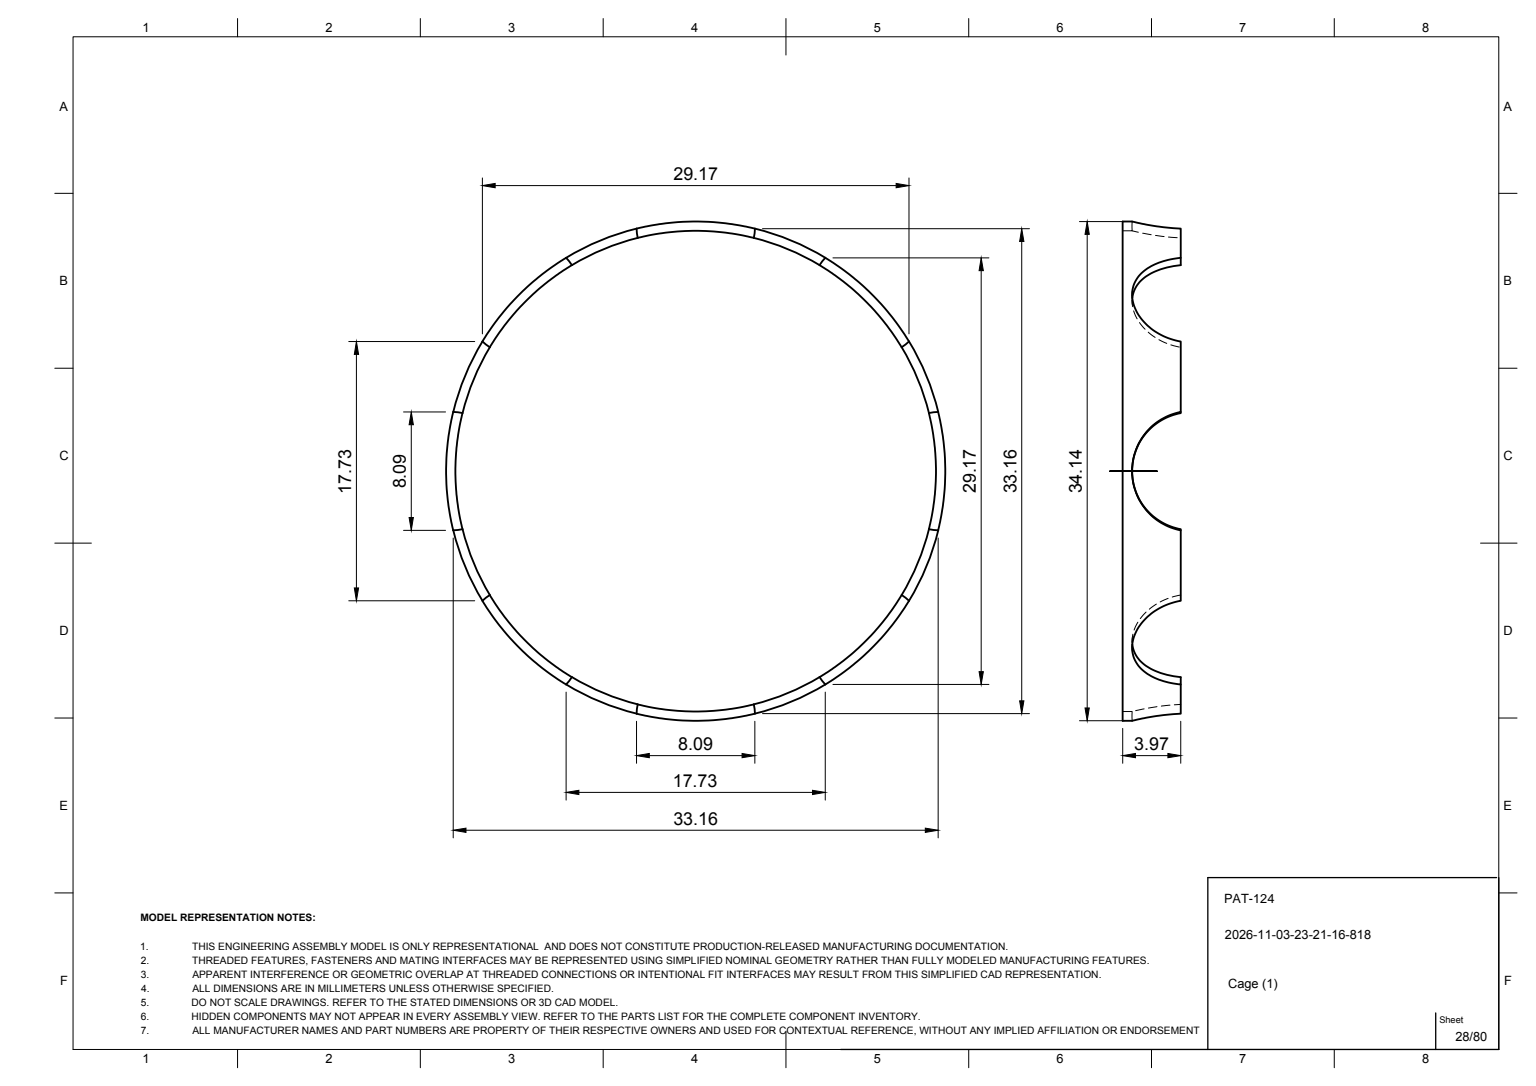
ISO-10303-21;
HEADER;
/* Generated by software containing ST-Developer
 * from STEP Tools, Inc. (www.steptools.com) 
 */

FILE_DESCRIPTION(
/* description */ ('XY cross-slide table'),
/* implementation_level */ '2;1');

FILE_NAME(
/* name */ 'Cage (1).step',
/* time_stamp */ '2026-10-28T03:22:46-07:00',
/* author */ (''),
/* organization */ (''),
/* preprocessor_version */ 'ST-DEVELOPER v20.2',
/* originating_system */ 'Autodesk Translation Framework v15.17.0.0',
/* authorisation */ '');

FILE_SCHEMA (('AUTOMOTIVE_DESIGN { 1 0 10303 214 3 1 1 }'));
ENDSEC;

DATA;
#10=MECHANICAL_DESIGN_GEOMETRIC_PRESENTATION_REPRESENTATION('',(#1703),#62984);
#707=B_SPLINE_CURVE_WITH_KNOTS('',3,(#34204,#34205,#34206,#34207,#34208,
#34209,#34210,#34211,#34212,#34213,#34214,#34215,#34216,#34217,#34218,#34219,
#34220,#34221,#34222,#34223,#34224,#34225),.UNSPECIFIED.,.F.,.F.,(4,2,2,
2,2,2,2,2,2,2,4),(0.0789094028588958,0.210573405340968,0.315860108011452,
0.421146810681936,0.522142632548711,0.623138454415485,0.72413427628226,
0.825130098149035,0.930416800819519,1.03570350349,1.16736750597208),
 .UNSPECIFIED.);
#708=B_SPLINE_CURVE_WITH_KNOTS('',3,(#34229,#34230,#34231,#34232,#34233,
#34234,#34235,#34236,#34237,#34238,#34239,#34240,#34241,#34242,#34243,#34244,
#34245,#34246,#34247,#34248,#34249,#34250),.UNSPECIFIED.,.F.,.F.,(4,2,2,
2,2,2,2,2,2,2,4),(0.0774793363974613,0.142088896491891,0.284177792983782,
0.411119756996526,0.514392970548519,0.617666184100513,0.720939397652506,
0.8242126112045,0.951154575217244,1.09324347170913,1.15785303180356),
 .UNSPECIFIED.);
#709=B_SPLINE_CURVE_WITH_KNOTS('',3,(#34256,#34257,#34258,#34259,#34260,
#34261,#34262,#34263,#34264,#34265,#34266,#34267,#34268,#34269,#34270,#34271,
#34272,#34273,#34274,#34275,#34276,#34277),.UNSPECIFIED.,.F.,.F.,(4,2,2,
2,2,2,2,2,2,2,4),(0.0774793363974613,0.142088896491891,0.284177792983782,
0.411119756996525,0.514392970548519,0.617666184100513,0.720939397652506,
0.8242126112045,0.951154575217243,1.09324347170913,1.15785303180356),
 .UNSPECIFIED.);
#710=B_SPLINE_CURVE_WITH_KNOTS('',3,(#34281,#34282,#34283,#34284,#34285,
#34286,#34287,#34288,#34289,#34290,#34291,#34292,#34293,#34294,#34295,#34296,
#34297,#34298,#34299,#34300,#34301,#34302),.UNSPECIFIED.,.F.,.F.,(4,2,2,
2,2,2,2,2,2,2,4),(0.0774793363974614,0.142088896491891,0.284177792983781,
0.411119756996525,0.514392970548519,0.617666184100512,0.720939397652506,
0.824212611204499,0.951154575217243,1.09324347170913,1.15785303180356),
 .UNSPECIFIED.);
#711=B_SPLINE_CURVE_WITH_KNOTS('',3,(#34306,#34307,#34308,#34309,#34310,
#34311,#34312,#34313,#34314,#34315,#34316,#34317),.UNSPECIFIED.,.F.,.F.,
(4,2,2,2,2,4),(0.0774793363974613,0.142088896491891,0.284177792983781,0.411119756996525,
0.514392970548519,0.617666184100512),.UNSPECIFIED.);
#712=B_SPLINE_CURVE_WITH_KNOTS('',3,(#34322,#34323,#34324,#34325,#34326,
#34327,#34328,#34329,#34330,#34331,#34332,#34333),.UNSPECIFIED.,.F.,.F.,
(4,2,2,2,2,4),(0.617666184100512,0.720939397652506,0.824212611204499,0.951154575217243,
1.09324347170913,1.15785303180356),.UNSPECIFIED.);
#713=B_SPLINE_CURVE_WITH_KNOTS('',3,(#34337,#34338,#34339,#34340,#34341,
#34342,#34343,#34344,#34345,#34346,#34347,#34348,#34349,#34350,#34351,#34352,
#34353,#34354,#34355,#34356,#34357,#34358),.UNSPECIFIED.,.F.,.F.,(4,2,2,
2,2,2,2,2,2,2,4),(0.0774793363974613,0.142088896491891,0.284177792983782,
0.411119756996526,0.514392970548519,0.617666184100513,0.720939397652507,
0.8242126112045,0.951154575217245,1.09324347170914,1.15785303180356),
 .UNSPECIFIED.);
#714=B_SPLINE_CURVE_WITH_KNOTS('',3,(#34362,#34363,#34364,#34365,#34366,
#34367,#34368,#34369,#34370,#34371,#34372,#34373,#34374,#34375,#34376,#34377,
#34378,#34379,#34380,#34381,#34382,#34383),.UNSPECIFIED.,.F.,.F.,(4,2,2,
2,2,2,2,2,2,2,4),(0.0774793363974613,0.142088896491891,0.284177792983782,
0.411119756996526,0.514392970548519,0.617666184100513,0.720939397652506,
0.824212611204499,0.951154575217243,1.09324347170913,1.15785303180356),
 .UNSPECIFIED.);
#715=B_SPLINE_CURVE_WITH_KNOTS('',3,(#34387,#34388,#34389,#34390,#34391,
#34392,#34393,#34394,#34395,#34396,#34397,#34398,#34399,#34400,#34401,#34402,
#34403,#34404,#34405,#34406,#34407,#34408),.UNSPECIFIED.,.F.,.F.,(4,2,2,
2,2,2,2,2,2,2,4),(0.0774793363974613,0.142088896491891,0.284177792983782,
0.411119756996526,0.514392970548519,0.617666184100513,0.720939397652506,
0.8242126112045,0.951154575217244,1.09324347170913,1.15785303180356),
 .UNSPECIFIED.);
#716=B_SPLINE_CURVE_WITH_KNOTS('',3,(#34412,#34413,#34414,#34415,#34416,
#34417,#34418,#34419,#34420,#34421,#34422,#34423,#34424,#34425,#34426,#34427,
#34428,#34429,#34430,#34431,#34432,#34433),.UNSPECIFIED.,.F.,.F.,(4,2,2,
2,2,2,2,2,2,2,4),(0.0774793363974613,0.142088896491891,0.284177792983782,
0.411119756996526,0.514392970548519,0.617666184100513,0.720939397652506,
0.8242126112045,0.951154575217243,1.09324347170913,1.15785303180356),
 .UNSPECIFIED.);
#717=B_SPLINE_CURVE_WITH_KNOTS('',3,(#34441,#34442,#34443,#34444,#34445,
#34446,#34447,#34448,#34449,#34450,#34451,#34452,#34453,#34454,#34455,#34456,
#34457,#34458,#34459,#34460,#34461,#34462),.UNSPECIFIED.,.F.,.F.,(4,2,2,
2,2,2,2,2,2,2,4),(0.0789094028588958,0.210573405340968,0.315860108011452,
0.421146810681936,0.522142632548711,0.623138454415485,0.72413427628226,
0.825130098149035,0.930416800819519,1.03570350349,1.16736750597208),
 .UNSPECIFIED.);
#718=B_SPLINE_CURVE_WITH_KNOTS('',3,(#34470,#34471,#34472,#34473,#34474,
#34475,#34476,#34477,#34478,#34479,#34480,#34481,#34482,#34483,#34484,#34485,
#34486,#34487,#34488,#34489,#34490,#34491),.UNSPECIFIED.,.F.,.F.,(4,2,2,
2,2,2,2,2,2,2,4),(0.0789094028588958,0.210573405340969,0.315860108011453,
0.421146810681937,0.522142632548712,0.623138454415486,0.724134276282261,
0.825130098149035,0.930416800819519,1.03570350349,1.16736750597208),
 .UNSPECIFIED.);
#719=B_SPLINE_CURVE_WITH_KNOTS('',3,(#34500,#34501,#34502,#34503,#34504,
#34505,#34506,#34507,#34508,#34509,#34510,#34511),.UNSPECIFIED.,.F.,.F.,
(4,2,2,2,2,4),(0.0789094028588958,0.210573405340968,0.315860108011452,0.421146810681937,
0.522142632548711,0.623138454415486),.UNSPECIFIED.);
#720=B_SPLINE_CURVE_WITH_KNOTS('',3,(#34513,#34514,#34515,#34516,#34517,
#34518,#34519,#34520,#34521,#34522,#34523,#34524),.UNSPECIFIED.,.F.,.F.,
(4,2,2,2,2,4),(0.623138454415486,0.72413427628226,0.825130098149035,0.930416800819519,
1.03570350349,1.16736750597208),.UNSPECIFIED.);
#721=B_SPLINE_CURVE_WITH_KNOTS('',3,(#34531,#34532,#34533,#34534,#34535,
#34536,#34537,#34538,#34539,#34540,#34541,#34542,#34543,#34544,#34545,#34546,
#34547,#34548,#34549,#34550,#34551,#34552),.UNSPECIFIED.,.F.,.F.,(4,2,2,
2,2,2,2,2,2,2,4),(0.0789094028588958,0.210573405340968,0.315860108011452,
0.421146810681936,0.522142632548711,0.623138454415486,0.72413427628226,
0.825130098149035,0.930416800819519,1.03570350349,1.16736750597208),
 .UNSPECIFIED.);
#722=B_SPLINE_CURVE_WITH_KNOTS('',3,(#34560,#34561,#34562,#34563,#34564,
#34565,#34566,#34567,#34568,#34569,#34570,#34571,#34572,#34573,#34574,#34575,
#34576,#34577,#34578,#34579,#34580,#34581),.UNSPECIFIED.,.F.,.F.,(4,2,2,
2,2,2,2,2,2,2,4),(0.0789094028588957,0.210573405340968,0.315860108011452,
0.421146810681936,0.522142632548711,0.623138454415485,0.72413427628226,
0.825130098149035,0.930416800819519,1.03570350349,1.16736750597207),
 .UNSPECIFIED.);
#723=B_SPLINE_CURVE_WITH_KNOTS('',3,(#34589,#34590,#34591,#34592,#34593,
#34594,#34595,#34596,#34597,#34598,#34599,#34600,#34601,#34602,#34603,#34604,
#34605,#34606,#34607,#34608,#34609,#34610),.UNSPECIFIED.,.F.,.F.,(4,2,2,
2,2,2,2,2,2,2,4),(0.0789094028588958,0.210573405340968,0.315860108011452,
0.421146810681936,0.522142632548711,0.623138454415486,0.72413427628226,
0.825130098149035,0.930416800819519,1.03570350349,1.16736750597208),
 .UNSPECIFIED.);
#724=B_SPLINE_CURVE_WITH_KNOTS('',3,(#34619,#34620,#34621,#34622,#34623,
#34624,#34625,#34626,#34627,#34628,#34629,#34630,#34631,#34632,#34633,#34634,
#34635,#34636,#34637,#34638,#34639,#34640),.UNSPECIFIED.,.F.,.F.,(4,2,2,
2,2,2,2,2,2,2,4),(0.0789094028588958,0.210573405340968,0.315860108011452,
0.421146810681936,0.522142632548711,0.623138454415485,0.72413427628226,
0.825130098149035,0.930416800819519,1.03570350349,1.16736750597208),
 .UNSPECIFIED.);
#1403=SPHERICAL_SURFACE('',#24472,0.412776);
#1404=SPHERICAL_SURFACE('',#24488,0.412776);
#1405=SPHERICAL_SURFACE('',#24493,0.412776);
#1406=SPHERICAL_SURFACE('',#24498,0.412776);
#1407=SPHERICAL_SURFACE('',#24503,0.412776);
#1408=SPHERICAL_SURFACE('',#24508,0.412776);
#1409=SPHERICAL_SURFACE('',#24513,0.412776);
#1410=SPHERICAL_SURFACE('',#24521,0.412776);
#1523=SHAPE_REPRESENTATION_RELATIONSHIP('SRR','None',#63373,#1606);
#1606=ADVANCED_BREP_SHAPE_REPRESENTATION('',(#1816),#62910);
#1703=STYLED_ITEM('',(#63912),#1816);
#1816=MANIFOLD_SOLID_BREP('Continuous crown cage',#22997);
#1996=FACE_BOUND('',#4529,.T.);
#2401=PLANE('',#24485);
#2402=PLANE('',#24490);
#2403=PLANE('',#24495);
#2404=PLANE('',#24500);
#2405=PLANE('',#24505);
#2406=PLANE('',#24510);
#2407=PLANE('',#24519);
#2408=PLANE('',#24523);
#2409=PLANE('',#24524);
#3088=FACE_OUTER_BOUND('',#4511,.T.);
#3089=FACE_OUTER_BOUND('',#4512,.T.);
#3090=FACE_OUTER_BOUND('',#4513,.T.);
#3091=FACE_OUTER_BOUND('',#4514,.T.);
#3092=FACE_OUTER_BOUND('',#4515,.T.);
#3093=FACE_OUTER_BOUND('',#4516,.T.);
#3094=FACE_OUTER_BOUND('',#4517,.T.);
#3095=FACE_OUTER_BOUND('',#4518,.T.);
#3096=FACE_OUTER_BOUND('',#4519,.T.);
#3097=FACE_OUTER_BOUND('',#4520,.T.);
#3098=FACE_OUTER_BOUND('',#4521,.T.);
#3099=FACE_OUTER_BOUND('',#4522,.T.);
#3100=FACE_OUTER_BOUND('',#4523,.T.);
#3101=FACE_OUTER_BOUND('',#4524,.T.);
#3102=FACE_OUTER_BOUND('',#4525,.T.);
#3103=FACE_OUTER_BOUND('',#4526,.T.);
#3104=FACE_OUTER_BOUND('',#4527,.T.);
#3105=FACE_OUTER_BOUND('',#4528,.T.);
#3106=FACE_OUTER_BOUND('',#4530,.T.);
#4511=EDGE_LOOP('',(#15832,#15833,#15834,#15835));
#4512=EDGE_LOOP('',(#15836,#15837,#15838,#15839,#15840,#15841,#15842,#15843,
#15844,#15845,#15846,#15847,#15848,#15849,#15850,#15851,#15852,#15853,#15854,
#15855));
#4513=EDGE_LOOP('',(#15856,#15857,#15858,#15859));
#4514=EDGE_LOOP('',(#15860,#15861,#15862,#15863));
#4515=EDGE_LOOP('',(#15864,#15865,#15866,#15867));
#4516=EDGE_LOOP('',(#15868,#15869,#15870,#15871));
#4517=EDGE_LOOP('',(#15872,#15873,#15874,#15875));
#4518=EDGE_LOOP('',(#15876,#15877,#15878,#15879,#15880,#15881));
#4519=EDGE_LOOP('',(#15882,#15883,#15884,#15885));
#4520=EDGE_LOOP('',(#15886,#15887,#15888,#15889));
#4521=EDGE_LOOP('',(#15890,#15891,#15892,#15893));
#4522=EDGE_LOOP('',(#15894,#15895,#15896,#15897));
#4523=EDGE_LOOP('',(#15898,#15899,#15900,#15901));
#4524=EDGE_LOOP('',(#15902,#15903,#15904,#15905));
#4525=EDGE_LOOP('',(#15906,#15907,#15908,#15909,#15910,#15911,#15912,#15913,
#15914,#15915,#15916,#15917,#15918,#15919,#15920,#15921,#15922,#15923,#15924,
#15925));
#4526=EDGE_LOOP('',(#15926,#15927,#15928,#15929));
#4527=EDGE_LOOP('',(#15930,#15931,#15932,#15933));
#4528=EDGE_LOOP('',(#15934));
#4529=EDGE_LOOP('',(#15935));
#4530=EDGE_LOOP('',(#15936,#15937,#15938,#15939));
#6133=LINE('',#34319,#7620);
#6134=LINE('',#34615,#7621);
#7620=VECTOR('',#27646,1.706752);
#7621=VECTOR('',#27723,1.643248);
#9103=CIRCLE('',#24473,0.405071403305639);
#9104=CIRCLE('',#24474,0.405071403305639);
#9105=CIRCLE('',#24476,1.706752);
#9106=CIRCLE('',#24477,1.706752);
#9107=CIRCLE('',#24478,1.706752);
#9108=CIRCLE('',#24479,1.706752);
#9109=CIRCLE('',#24480,1.706752);
#9110=CIRCLE('',#24481,1.706752);
#9111=CIRCLE('',#24482,1.706752);
#9112=CIRCLE('',#24483,1.706752);
#9113=CIRCLE('',#24484,1.706752);
#9114=CIRCLE('',#24486,1.643248);
#9115=CIRCLE('',#24487,0.405071403305639);
#9116=CIRCLE('',#24489,0.405071403305639);
#9117=CIRCLE('',#24491,1.643248);
#9118=CIRCLE('',#24492,0.405071403305639);
#9119=CIRCLE('',#24494,0.405071403305639);
#9120=CIRCLE('',#24496,1.643248);
#9121=CIRCLE('',#24497,0.405071403305639);
#9122=CIRCLE('',#24499,0.405071403305639);
#9123=CIRCLE('',#24501,1.643248);
#9124=CIRCLE('',#24502,0.405071403305639);
#9125=CIRCLE('',#24504,0.405071403305639);
#9126=CIRCLE('',#24506,1.643248);
#9127=CIRCLE('',#24507,0.405071403305639);
#9128=CIRCLE('',#24509,0.405071403305639);
#9129=CIRCLE('',#24511,1.643248);
#9130=CIRCLE('',#24512,0.405071403305639);
#9131=CIRCLE('',#24514,0.405071403305639);
#9132=CIRCLE('',#24516,1.643248);
#9133=CIRCLE('',#24517,1.643248);
#9134=CIRCLE('',#24518,1.643248);
#9135=CIRCLE('',#24520,0.405071403305639);
#9136=CIRCLE('',#24522,0.405071403305639);
#10097=VERTEX_POINT('',#34202);
#10098=VERTEX_POINT('',#34203);
#10099=VERTEX_POINT('',#34226);
#10100=VERTEX_POINT('',#34228);
#10101=VERTEX_POINT('',#34253);
#10102=VERTEX_POINT('',#34255);
#10103=VERTEX_POINT('',#34278);
#10104=VERTEX_POINT('',#34280);
#10105=VERTEX_POINT('',#34303);
#10106=VERTEX_POINT('',#34305);
#10107=VERTEX_POINT('',#34318);
#10108=VERTEX_POINT('',#34321);
#10109=VERTEX_POINT('',#34334);
#10110=VERTEX_POINT('',#34336);
#10111=VERTEX_POINT('',#34359);
#10112=VERTEX_POINT('',#34361);
#10113=VERTEX_POINT('',#34384);
#10114=VERTEX_POINT('',#34386);
#10115=VERTEX_POINT('',#34409);
#10116=VERTEX_POINT('',#34411);
#10117=VERTEX_POINT('',#34436);
#10118=VERTEX_POINT('',#34440);
#10119=VERTEX_POINT('',#34465);
#10120=VERTEX_POINT('',#34469);
#10121=VERTEX_POINT('',#34494);
#10122=VERTEX_POINT('',#34498);
#10123=VERTEX_POINT('',#34499);
#10124=VERTEX_POINT('',#34526);
#10125=VERTEX_POINT('',#34530);
#10126=VERTEX_POINT('',#34555);
#10127=VERTEX_POINT('',#34559);
#10128=VERTEX_POINT('',#34584);
#10129=VERTEX_POINT('',#34588);
#10130=VERTEX_POINT('',#34613);
#10131=VERTEX_POINT('',#34616);
#10132=VERTEX_POINT('',#34618);
#12300=EDGE_CURVE('',#10097,#10098,#707,.T.);
#12301=EDGE_CURVE('',#10099,#10097,#9103,.T.);
#12302=EDGE_CURVE('',#10100,#10099,#708,.T.);
#12303=EDGE_CURVE('',#10098,#10100,#9104,.T.);
#12304=EDGE_CURVE('',#10101,#10099,#9105,.T.);
#12305=EDGE_CURVE('',#10101,#10102,#709,.T.);
#12306=EDGE_CURVE('',#10103,#10102,#9106,.T.);
#12307=EDGE_CURVE('',#10103,#10104,#710,.T.);
#12308=EDGE_CURVE('',#10105,#10104,#9107,.T.);
#12309=EDGE_CURVE('',#10105,#10106,#711,.T.);
#12310=EDGE_CURVE('',#10106,#10107,#6133,.T.);
#12311=EDGE_CURVE('',#10107,#10107,#9108,.T.);
#12312=EDGE_CURVE('',#10106,#10108,#712,.T.);
#12313=EDGE_CURVE('',#10109,#10108,#9109,.T.);
#12314=EDGE_CURVE('',#10109,#10110,#713,.T.);
#12315=EDGE_CURVE('',#10111,#10110,#9110,.T.);
#12316=EDGE_CURVE('',#10111,#10112,#714,.T.);
#12317=EDGE_CURVE('',#10113,#10112,#9111,.T.);
#12318=EDGE_CURVE('',#10113,#10114,#715,.T.);
#12319=EDGE_CURVE('',#10115,#10114,#9112,.T.);
#12320=EDGE_CURVE('',#10115,#10116,#716,.T.);
#12321=EDGE_CURVE('',#10100,#10116,#9113,.T.);
#12322=EDGE_CURVE('',#10097,#10117,#9114,.T.);
#12323=EDGE_CURVE('',#10117,#10101,#9115,.T.);
#12324=EDGE_CURVE('',#10118,#10117,#717,.T.);
#12325=EDGE_CURVE('',#10102,#10118,#9116,.T.);
#12326=EDGE_CURVE('',#10118,#10119,#9117,.T.);
#12327=EDGE_CURVE('',#10119,#10103,#9118,.T.);
#12328=EDGE_CURVE('',#10120,#10119,#718,.T.);
#12329=EDGE_CURVE('',#10104,#10120,#9119,.T.);
#12330=EDGE_CURVE('',#10120,#10121,#9120,.T.);
#12331=EDGE_CURVE('',#10121,#10105,#9121,.T.);
#12332=EDGE_CURVE('',#10122,#10123,#719,.T.);
#12333=EDGE_CURVE('',#10108,#10122,#9122,.T.);
#12334=EDGE_CURVE('',#10123,#10121,#720,.T.);
#12335=EDGE_CURVE('',#10122,#10124,#9123,.T.);
#12336=EDGE_CURVE('',#10124,#10109,#9124,.T.);
#12337=EDGE_CURVE('',#10125,#10124,#721,.T.);
#12338=EDGE_CURVE('',#10110,#10125,#9125,.T.);
#12339=EDGE_CURVE('',#10125,#10126,#9126,.T.);
#12340=EDGE_CURVE('',#10126,#10111,#9127,.T.);
#12341=EDGE_CURVE('',#10127,#10126,#722,.T.);
#12342=EDGE_CURVE('',#10112,#10127,#9128,.T.);
#12343=EDGE_CURVE('',#10127,#10128,#9129,.T.);
#12344=EDGE_CURVE('',#10128,#10113,#9130,.T.);
#12345=EDGE_CURVE('',#10129,#10128,#723,.T.);
#12346=EDGE_CURVE('',#10114,#10129,#9131,.T.);
#12347=EDGE_CURVE('',#10130,#10130,#9132,.T.);
#12348=EDGE_CURVE('',#10130,#10123,#6134,.T.);
#12349=EDGE_CURVE('',#10131,#10098,#9133,.T.);
#12350=EDGE_CURVE('',#10131,#10132,#724,.T.);
#12351=EDGE_CURVE('',#10129,#10132,#9134,.T.);
#12352=EDGE_CURVE('',#10116,#10131,#9135,.T.);
#12353=EDGE_CURVE('',#10132,#10115,#9136,.T.);
#15832=ORIENTED_EDGE('',*,*,#12300,.F.);
#15833=ORIENTED_EDGE('',*,*,#12301,.F.);
#15834=ORIENTED_EDGE('',*,*,#12302,.F.);
#15835=ORIENTED_EDGE('',*,*,#12303,.F.);
#15836=ORIENTED_EDGE('',*,*,#12302,.T.);
#15837=ORIENTED_EDGE('',*,*,#12304,.F.);
#15838=ORIENTED_EDGE('',*,*,#12305,.T.);
#15839=ORIENTED_EDGE('',*,*,#12306,.F.);
#15840=ORIENTED_EDGE('',*,*,#12307,.T.);
#15841=ORIENTED_EDGE('',*,*,#12308,.F.);
#15842=ORIENTED_EDGE('',*,*,#12309,.T.);
#15843=ORIENTED_EDGE('',*,*,#12310,.T.);
#15844=ORIENTED_EDGE('',*,*,#12311,.F.);
#15845=ORIENTED_EDGE('',*,*,#12310,.F.);
#15846=ORIENTED_EDGE('',*,*,#12312,.T.);
#15847=ORIENTED_EDGE('',*,*,#12313,.F.);
#15848=ORIENTED_EDGE('',*,*,#12314,.T.);
#15849=ORIENTED_EDGE('',*,*,#12315,.F.);
#15850=ORIENTED_EDGE('',*,*,#12316,.T.);
#15851=ORIENTED_EDGE('',*,*,#12317,.F.);
#15852=ORIENTED_EDGE('',*,*,#12318,.T.);
#15853=ORIENTED_EDGE('',*,*,#12319,.F.);
#15854=ORIENTED_EDGE('',*,*,#12320,.T.);
#15855=ORIENTED_EDGE('',*,*,#12321,.F.);
#15856=ORIENTED_EDGE('',*,*,#12301,.T.);
#15857=ORIENTED_EDGE('',*,*,#12322,.T.);
#15858=ORIENTED_EDGE('',*,*,#12323,.T.);
#15859=ORIENTED_EDGE('',*,*,#12304,.T.);
#15860=ORIENTED_EDGE('',*,*,#12324,.F.);
#15861=ORIENTED_EDGE('',*,*,#12325,.F.);
#15862=ORIENTED_EDGE('',*,*,#12305,.F.);
#15863=ORIENTED_EDGE('',*,*,#12323,.F.);
#15864=ORIENTED_EDGE('',*,*,#12325,.T.);
#15865=ORIENTED_EDGE('',*,*,#12326,.T.);
#15866=ORIENTED_EDGE('',*,*,#12327,.T.);
#15867=ORIENTED_EDGE('',*,*,#12306,.T.);
#15868=ORIENTED_EDGE('',*,*,#12328,.F.);
#15869=ORIENTED_EDGE('',*,*,#12329,.F.);
#15870=ORIENTED_EDGE('',*,*,#12307,.F.);
#15871=ORIENTED_EDGE('',*,*,#12327,.F.);
#15872=ORIENTED_EDGE('',*,*,#12329,.T.);
#15873=ORIENTED_EDGE('',*,*,#12330,.T.);
#15874=ORIENTED_EDGE('',*,*,#12331,.T.);
#15875=ORIENTED_EDGE('',*,*,#12308,.T.);
#15876=ORIENTED_EDGE('',*,*,#12332,.F.);
#15877=ORIENTED_EDGE('',*,*,#12333,.F.);
#15878=ORIENTED_EDGE('',*,*,#12312,.F.);
#15879=ORIENTED_EDGE('',*,*,#12309,.F.);
#15880=ORIENTED_EDGE('',*,*,#12331,.F.);
#15881=ORIENTED_EDGE('',*,*,#12334,.F.);
#15882=ORIENTED_EDGE('',*,*,#12333,.T.);
#15883=ORIENTED_EDGE('',*,*,#12335,.T.);
#15884=ORIENTED_EDGE('',*,*,#12336,.T.);
#15885=ORIENTED_EDGE('',*,*,#12313,.T.);
#15886=ORIENTED_EDGE('',*,*,#12337,.F.);
#15887=ORIENTED_EDGE('',*,*,#12338,.F.);
#15888=ORIENTED_EDGE('',*,*,#12314,.F.);
#15889=ORIENTED_EDGE('',*,*,#12336,.F.);
#15890=ORIENTED_EDGE('',*,*,#12338,.T.);
#15891=ORIENTED_EDGE('',*,*,#12339,.T.);
#15892=ORIENTED_EDGE('',*,*,#12340,.T.);
#15893=ORIENTED_EDGE('',*,*,#12315,.T.);
#15894=ORIENTED_EDGE('',*,*,#12341,.F.);
#15895=ORIENTED_EDGE('',*,*,#12342,.F.);
#15896=ORIENTED_EDGE('',*,*,#12316,.F.);
#15897=ORIENTED_EDGE('',*,*,#12340,.F.);
#15898=ORIENTED_EDGE('',*,*,#12342,.T.);
#15899=ORIENTED_EDGE('',*,*,#12343,.T.);
#15900=ORIENTED_EDGE('',*,*,#12344,.T.);
#15901=ORIENTED_EDGE('',*,*,#12317,.T.);
#15902=ORIENTED_EDGE('',*,*,#12318,.F.);
#15903=ORIENTED_EDGE('',*,*,#12344,.F.);
#15904=ORIENTED_EDGE('',*,*,#12345,.F.);
#15905=ORIENTED_EDGE('',*,*,#12346,.F.);
#15906=ORIENTED_EDGE('',*,*,#12347,.F.);
#15907=ORIENTED_EDGE('',*,*,#12348,.T.);
#15908=ORIENTED_EDGE('',*,*,#12334,.T.);
#15909=ORIENTED_EDGE('',*,*,#12330,.F.);
#15910=ORIENTED_EDGE('',*,*,#12328,.T.);
#15911=ORIENTED_EDGE('',*,*,#12326,.F.);
#15912=ORIENTED_EDGE('',*,*,#12324,.T.);
#15913=ORIENTED_EDGE('',*,*,#12322,.F.);
#15914=ORIENTED_EDGE('',*,*,#12300,.T.);
#15915=ORIENTED_EDGE('',*,*,#12349,.F.);
#15916=ORIENTED_EDGE('',*,*,#12350,.T.);
#15917=ORIENTED_EDGE('',*,*,#12351,.F.);
#15918=ORIENTED_EDGE('',*,*,#12345,.T.);
#15919=ORIENTED_EDGE('',*,*,#12343,.F.);
#15920=ORIENTED_EDGE('',*,*,#12341,.T.);
#15921=ORIENTED_EDGE('',*,*,#12339,.F.);
#15922=ORIENTED_EDGE('',*,*,#12337,.T.);
#15923=ORIENTED_EDGE('',*,*,#12335,.F.);
#15924=ORIENTED_EDGE('',*,*,#12332,.T.);
#15925=ORIENTED_EDGE('',*,*,#12348,.F.);
#15926=ORIENTED_EDGE('',*,*,#12303,.T.);
#15927=ORIENTED_EDGE('',*,*,#12321,.T.);
#15928=ORIENTED_EDGE('',*,*,#12352,.T.);
#15929=ORIENTED_EDGE('',*,*,#12349,.T.);
#15930=ORIENTED_EDGE('',*,*,#12320,.F.);
#15931=ORIENTED_EDGE('',*,*,#12353,.F.);
#15932=ORIENTED_EDGE('',*,*,#12350,.F.);
#15933=ORIENTED_EDGE('',*,*,#12352,.F.);
#15934=ORIENTED_EDGE('',*,*,#12311,.T.);
#15935=ORIENTED_EDGE('',*,*,#12347,.T.);
#15936=ORIENTED_EDGE('',*,*,#12346,.T.);
#15937=ORIENTED_EDGE('',*,*,#12351,.T.);
#15938=ORIENTED_EDGE('',*,*,#12353,.T.);
#15939=ORIENTED_EDGE('',*,*,#12319,.T.);
#21120=CYLINDRICAL_SURFACE('',#24475,1.706752);
#21121=CYLINDRICAL_SURFACE('',#24515,1.643248);
#21869=ADVANCED_FACE('',(#3088),#1403,.F.);
#21870=ADVANCED_FACE('',(#3089),#21120,.T.);
#21871=ADVANCED_FACE('',(#3090),#2401,.T.);
#21872=ADVANCED_FACE('',(#3091),#1404,.F.);
#21873=ADVANCED_FACE('',(#3092),#2402,.T.);
#21874=ADVANCED_FACE('',(#3093),#1405,.F.);
#21875=ADVANCED_FACE('',(#3094),#2403,.T.);
#21876=ADVANCED_FACE('',(#3095),#1406,.F.);
#21877=ADVANCED_FACE('',(#3096),#2404,.T.);
#21878=ADVANCED_FACE('',(#3097),#1407,.F.);
#21879=ADVANCED_FACE('',(#3098),#2405,.T.);
#21880=ADVANCED_FACE('',(#3099),#1408,.F.);
#21881=ADVANCED_FACE('',(#3100),#2406,.T.);
#21882=ADVANCED_FACE('',(#3101),#1409,.F.);
#21883=ADVANCED_FACE('',(#3102),#21121,.F.);
#21884=ADVANCED_FACE('',(#3103),#2407,.T.);
#21885=ADVANCED_FACE('',(#3104),#1410,.F.);
#21886=ADVANCED_FACE('',(#3105,#1996),#2408,.T.);
#21887=ADVANCED_FACE('',(#3106),#2409,.T.);
#22997=CLOSED_SHELL('',(#21869,#21870,#21871,#21872,#21873,#21874,#21875,
#21876,#21877,#21878,#21879,#21880,#21881,#21882,#21883,#21884,#21885,#21886,
#21887));
#24471=AXIS2_PLACEMENT_3D('',#34200,#27630,#27631);
#24472=AXIS2_PLACEMENT_3D('',#34201,#27632,#27633);
#24473=AXIS2_PLACEMENT_3D('',#34227,#27634,#27635);
#24474=AXIS2_PLACEMENT_3D('',#34251,#27636,#27637);
#24475=AXIS2_PLACEMENT_3D('',#34252,#27638,#27639);
#24476=AXIS2_PLACEMENT_3D('',#34254,#27640,#27641);
#24477=AXIS2_PLACEMENT_3D('',#34279,#27642,#27643);
#24478=AXIS2_PLACEMENT_3D('',#34304,#27644,#27645);
#24479=AXIS2_PLACEMENT_3D('',#34320,#27647,#27648);
#24480=AXIS2_PLACEMENT_3D('',#34335,#27649,#27650);
#24481=AXIS2_PLACEMENT_3D('',#34360,#27651,#27652);
#24482=AXIS2_PLACEMENT_3D('',#34385,#27653,#27654);
#24483=AXIS2_PLACEMENT_3D('',#34410,#27655,#27656);
#24484=AXIS2_PLACEMENT_3D('',#34434,#27657,#27658);
#24485=AXIS2_PLACEMENT_3D('',#34435,#27659,#27660);
#24486=AXIS2_PLACEMENT_3D('',#34437,#27661,#27662);
#24487=AXIS2_PLACEMENT_3D('',#34438,#27663,#27664);
#24488=AXIS2_PLACEMENT_3D('',#34439,#27665,#27666);
#24489=AXIS2_PLACEMENT_3D('',#34463,#27667,#27668);
#24490=AXIS2_PLACEMENT_3D('',#34464,#27669,#27670);
#24491=AXIS2_PLACEMENT_3D('',#34466,#27671,#27672);
#24492=AXIS2_PLACEMENT_3D('',#34467,#27673,#27674);
#24493=AXIS2_PLACEMENT_3D('',#34468,#27675,#27676);
#24494=AXIS2_PLACEMENT_3D('',#34492,#27677,#27678);
#24495=AXIS2_PLACEMENT_3D('',#34493,#27679,#27680);
#24496=AXIS2_PLACEMENT_3D('',#34495,#27681,#27682);
#24497=AXIS2_PLACEMENT_3D('',#34496,#27683,#27684);
#24498=AXIS2_PLACEMENT_3D('',#34497,#27685,#27686);
#24499=AXIS2_PLACEMENT_3D('',#34512,#27687,#27688);
#24500=AXIS2_PLACEMENT_3D('',#34525,#27689,#27690);
#24501=AXIS2_PLACEMENT_3D('',#34527,#27691,#27692);
#24502=AXIS2_PLACEMENT_3D('',#34528,#27693,#27694);
#24503=AXIS2_PLACEMENT_3D('',#34529,#27695,#27696);
#24504=AXIS2_PLACEMENT_3D('',#34553,#27697,#27698);
#24505=AXIS2_PLACEMENT_3D('',#34554,#27699,#27700);
#24506=AXIS2_PLACEMENT_3D('',#34556,#27701,#27702);
#24507=AXIS2_PLACEMENT_3D('',#34557,#27703,#27704);
#24508=AXIS2_PLACEMENT_3D('',#34558,#27705,#27706);
#24509=AXIS2_PLACEMENT_3D('',#34582,#27707,#27708);
#24510=AXIS2_PLACEMENT_3D('',#34583,#27709,#27710);
#24511=AXIS2_PLACEMENT_3D('',#34585,#27711,#27712);
#24512=AXIS2_PLACEMENT_3D('',#34586,#27713,#27714);
#24513=AXIS2_PLACEMENT_3D('',#34587,#27715,#27716);
#24514=AXIS2_PLACEMENT_3D('',#34611,#27717,#27718);
#24515=AXIS2_PLACEMENT_3D('',#34612,#27719,#27720);
#24516=AXIS2_PLACEMENT_3D('',#34614,#27721,#27722);
#24517=AXIS2_PLACEMENT_3D('',#34617,#27724,#27725);
#24518=AXIS2_PLACEMENT_3D('',#34641,#27726,#27727);
#24519=AXIS2_PLACEMENT_3D('',#34642,#27728,#27729);
#24520=AXIS2_PLACEMENT_3D('',#34643,#27730,#27731);
#24521=AXIS2_PLACEMENT_3D('',#34644,#27732,#27733);
#24522=AXIS2_PLACEMENT_3D('',#34645,#27734,#27735);
#24523=AXIS2_PLACEMENT_3D('',#34646,#27736,#27737);
#24524=AXIS2_PLACEMENT_3D('',#34647,#27738,#27739);
#27630=DIRECTION('axis',(0.,0.,1.));
#27631=DIRECTION('refdir',(1.,0.,0.));
#27632=DIRECTION('center_axis',(0.,0.,1.));
#27633=DIRECTION('ref_axis',(1.,0.,0.));
#27634=DIRECTION('center_axis',(0.,-1.,0.));
#27635=DIRECTION('ref_axis',(0.,0.,-1.));
#27636=DIRECTION('center_axis',(0.,-1.,0.));
#27637=DIRECTION('ref_axis',(0.,0.,-1.));
#27638=DIRECTION('center_axis',(0.,1.,0.));
#27639=DIRECTION('ref_axis',(1.,0.,0.));
#27640=DIRECTION('center_axis',(0.,1.,0.));
#27641=DIRECTION('ref_axis',(1.,0.,0.));
#27642=DIRECTION('center_axis',(0.,1.,0.));
#27643=DIRECTION('ref_axis',(1.,0.,0.));
#27644=DIRECTION('center_axis',(0.,1.,0.));
#27645=DIRECTION('ref_axis',(1.,0.,0.));
#27646=DIRECTION('',(0.,-1.,0.));
#27647=DIRECTION('center_axis',(0.,-1.,0.));
#27648=DIRECTION('ref_axis',(1.,0.,0.));
#27649=DIRECTION('center_axis',(0.,1.,0.));
#27650=DIRECTION('ref_axis',(1.,0.,0.));
#27651=DIRECTION('center_axis',(0.,1.,0.));
#27652=DIRECTION('ref_axis',(1.,0.,0.));
#27653=DIRECTION('center_axis',(0.,1.,0.));
#27654=DIRECTION('ref_axis',(1.,0.,0.));
#27655=DIRECTION('center_axis',(0.,1.,0.));
#27656=DIRECTION('ref_axis',(1.,0.,0.));
#27657=DIRECTION('center_axis',(0.,1.,0.));
#27658=DIRECTION('ref_axis',(1.,0.,0.));
#27659=DIRECTION('center_axis',(0.,1.,0.));
#27660=DIRECTION('ref_axis',(1.,0.,0.));
#27661=DIRECTION('center_axis',(0.,-1.,0.));
#27662=DIRECTION('ref_axis',(1.,0.,0.));
#27663=DIRECTION('center_axis',(0.,-1.,0.));
#27664=DIRECTION('ref_axis',(0.,0.,-1.));
#27665=DIRECTION('center_axis',(6.12323399573677E-17,0.,1.));
#27666=DIRECTION('ref_axis',(1.,0.,0.));
#27667=DIRECTION('center_axis',(0.,-1.,0.));
#27668=DIRECTION('ref_axis',(0.,0.,-1.));
#27669=DIRECTION('center_axis',(0.,1.,0.));
#27670=DIRECTION('ref_axis',(1.,0.,0.));
#27671=DIRECTION('center_axis',(0.,-1.,0.));
#27672=DIRECTION('ref_axis',(1.,0.,0.));
#27673=DIRECTION('center_axis',(0.,-1.,0.));
#27674=DIRECTION('ref_axis',(0.,0.,-1.));
#27675=DIRECTION('center_axis',(0.,0.,1.));
#27676=DIRECTION('ref_axis',(1.,0.,0.));
#27677=DIRECTION('center_axis',(0.,-1.,0.));
#27678=DIRECTION('ref_axis',(0.,0.,-1.));
#27679=DIRECTION('center_axis',(0.,1.,0.));
#27680=DIRECTION('ref_axis',(1.,0.,0.));
#27681=DIRECTION('center_axis',(0.,-1.,0.));
#27682=DIRECTION('ref_axis',(1.,0.,0.));
#27683=DIRECTION('center_axis',(0.,-1.,0.));
#27684=DIRECTION('ref_axis',(0.,0.,-1.));
#27685=DIRECTION('center_axis',(0.,0.,1.));
#27686=DIRECTION('ref_axis',(1.,0.,0.));
#27687=DIRECTION('center_axis',(0.,-1.,0.));
#27688=DIRECTION('ref_axis',(0.,0.,-1.));
#27689=DIRECTION('center_axis',(0.,1.,0.));
#27690=DIRECTION('ref_axis',(1.,0.,0.));
#27691=DIRECTION('center_axis',(0.,-1.,0.));
#27692=DIRECTION('ref_axis',(1.,0.,0.));
#27693=DIRECTION('center_axis',(0.,-1.,0.));
#27694=DIRECTION('ref_axis',(0.,0.,-1.));
#27695=DIRECTION('center_axis',(0.,0.,1.));
#27696=DIRECTION('ref_axis',(1.,0.,0.));
#27697=DIRECTION('center_axis',(0.,-1.,0.));
#27698=DIRECTION('ref_axis',(0.,0.,-1.));
#27699=DIRECTION('center_axis',(0.,1.,0.));
#27700=DIRECTION('ref_axis',(1.,0.,0.));
#27701=DIRECTION('center_axis',(0.,-1.,0.));
#27702=DIRECTION('ref_axis',(1.,0.,0.));
#27703=DIRECTION('center_axis',(0.,-1.,0.));
#27704=DIRECTION('ref_axis',(0.,0.,-1.));
#27705=DIRECTION('center_axis',(6.12323399573676E-17,0.,1.));
#27706=DIRECTION('ref_axis',(1.,0.,0.));
#27707=DIRECTION('center_axis',(0.,-1.,0.));
#27708=DIRECTION('ref_axis',(0.,0.,-1.));
#27709=DIRECTION('center_axis',(0.,1.,0.));
#27710=DIRECTION('ref_axis',(1.,0.,0.));
#27711=DIRECTION('center_axis',(0.,-1.,0.));
#27712=DIRECTION('ref_axis',(1.,0.,0.));
#27713=DIRECTION('center_axis',(0.,-1.,0.));
#27714=DIRECTION('ref_axis',(0.,0.,-1.));
#27715=DIRECTION('center_axis',(0.,0.,1.));
#27716=DIRECTION('ref_axis',(1.,0.,0.));
#27717=DIRECTION('center_axis',(0.,-1.,0.));
#27718=DIRECTION('ref_axis',(0.,0.,-1.));
#27719=DIRECTION('center_axis',(0.,1.,0.));
#27720=DIRECTION('ref_axis',(1.,0.,0.));
#27721=DIRECTION('center_axis',(0.,1.,0.));
#27722=DIRECTION('ref_axis',(1.,0.,0.));
#27723=DIRECTION('',(0.,1.,0.));
#27724=DIRECTION('center_axis',(0.,-1.,0.));
#27725=DIRECTION('ref_axis',(1.,0.,0.));
#27726=DIRECTION('center_axis',(0.,-1.,0.));
#27727=DIRECTION('ref_axis',(1.,0.,0.));
#27728=DIRECTION('center_axis',(0.,1.,0.));
#27729=DIRECTION('ref_axis',(1.,0.,0.));
#27730=DIRECTION('center_axis',(0.,-1.,0.));
#27731=DIRECTION('ref_axis',(0.,0.,-1.));
#27732=DIRECTION('center_axis',(0.,0.,1.));
#27733=DIRECTION('ref_axis',(1.,0.,0.));
#27734=DIRECTION('center_axis',(0.,-1.,0.));
#27735=DIRECTION('ref_axis',(0.,0.,-1.));
#27736=DIRECTION('center_axis',(0.,-1.,0.));
#27737=DIRECTION('ref_axis',(-1.,0.,0.));
#27738=DIRECTION('center_axis',(0.,1.,0.));
#27739=DIRECTION('ref_axis',(1.,0.,0.));
#34200=CARTESIAN_POINT('',(0.,0.,0.));
#34201=CARTESIAN_POINT('Origin',(1.18440385848747,0.,1.18440385848747));
#34202=CARTESIAN_POINT('',(0.846804978391753,-0.07938,1.40825612658882));
#34203=CARTESIAN_POINT('',(1.40825612658882,-0.07938,0.846804978391754));
#34204=CARTESIAN_POINT('Ctrl Pts',(0.846804978391752,-0.0793800000000001,
1.40825612658882));
#34205=CARTESIAN_POINT('Ctrl Pts',(0.854205272175554,-0.123401821157026,
1.40380622184538));
#34206=CARTESIAN_POINT('Ctrl Pts',(0.867957148219441,-0.166543350814306,
1.39550172959303));
#34207=CARTESIAN_POINT('Ctrl Pts',(0.902193646979982,-0.237231147975234,
1.3735491215176));
#34208=CARTESIAN_POINT('Ctrl Pts',(0.920778333482564,-0.266264900654909,
1.36127834356734));
#34209=CARTESIAN_POINT('Ctrl Pts',(0.962485392528369,-0.317195968905306,
1.33211611256184));
#34210=CARTESIAN_POINT('Ctrl Pts',(0.985600426557816,-0.33909093068465,
1.31521005565926));
#34211=CARTESIAN_POINT('Ctrl Pts',(1.03253285680459,-0.373586846396559,
1.27866649102984));
#34212=CARTESIAN_POINT('Ctrl Pts',(1.05871835910697,-0.388086240756494,
1.25722555095714));
#34213=CARTESIAN_POINT('Ctrl Pts',(1.11153475808518,-0.407068917407805,
1.2107812086231));
#34214=CARTESIAN_POINT('Ctrl Pts',(1.13814686046673,-0.411552957311693,
1.18575674747573));
#34215=CARTESIAN_POINT('Ctrl Pts',(1.18575674747573,-0.411552957311693,
1.13814686046673));
#34216=CARTESIAN_POINT('Ctrl Pts',(1.2107812086231,-0.407068917407805,1.11153475808518));
#34217=CARTESIAN_POINT('Ctrl Pts',(1.25722555095713,-0.388086240756494,
1.05871835910697));
#34218=CARTESIAN_POINT('Ctrl Pts',(1.27866649102984,-0.373586846396559,
1.03253285680459));
#34219=CARTESIAN_POINT('Ctrl Pts',(1.31521005565926,-0.33909093068465,0.985600426557816));
#34220=CARTESIAN_POINT('Ctrl Pts',(1.33211611256184,-0.317195968905306,
0.962485392528369));
#34221=CARTESIAN_POINT('Ctrl Pts',(1.36127834356734,-0.266264900654909,
0.920778333482565));
#34222=CARTESIAN_POINT('Ctrl Pts',(1.3735491215176,-0.237231147975234,0.902193646979983));
#34223=CARTESIAN_POINT('Ctrl Pts',(1.39550172959303,-0.166543350814306,
0.867957148219442));
#34224=CARTESIAN_POINT('Ctrl Pts',(1.40380622184538,-0.123401821157026,
0.854205272175555));
#34225=CARTESIAN_POINT('Ctrl Pts',(1.40825612658882,-0.0793800000000001,
0.846804978391753));
#34226=CARTESIAN_POINT('',(0.886256117232623,-0.07938,1.45861320581289));
#34227=CARTESIAN_POINT('Origin',(1.18440385848747,-0.07938,1.18440385848747));
#34228=CARTESIAN_POINT('',(1.45861320581289,-0.07938,0.886256117232624));
#34229=CARTESIAN_POINT('Ctrl Pts',(1.45861320581289,-0.0793800000000001,
0.886256117232623));
#34230=CARTESIAN_POINT('Ctrl Pts',(1.45630208793976,-0.101649918886749,
0.890059788636852));
#34231=CARTESIAN_POINT('Ctrl Pts',(1.45296717977858,-0.123823518623746,
0.895520212222107));
#34232=CARTESIAN_POINT('Ctrl Pts',(1.43904931717599,-0.192480977588836,
0.917859913453975));
#34233=CARTESIAN_POINT('Ctrl Pts',(1.4243271592157,-0.236152929235938,0.940896403863072));
#34234=CARTESIAN_POINT('Ctrl Pts',(1.39055359345152,-0.303141259068212,
0.990027513266106));
#34235=CARTESIAN_POINT('Ctrl Pts',(1.36743459453896,-0.335108247315849,
1.02199477007745));
#34236=CARTESIAN_POINT('Ctrl Pts',(1.32643091652006,-0.373243761060364,
1.07446535104584));
#34237=CARTESIAN_POINT('Ctrl Pts',(1.30441816675528,-0.387888272594439,
1.10126842659597));
#34238=CARTESIAN_POINT('Ctrl Pts',(1.25681160160691,-0.407041111792943,
1.15530234155453));
#34239=CARTESIAN_POINT('Ctrl Pts',(1.23119764287622,-0.411552957311693,
1.18251418313119));
#34240=CARTESIAN_POINT('Ctrl Pts',(1.18251418313119,-0.411552957311693,
1.23119764287622));
#34241=CARTESIAN_POINT('Ctrl Pts',(1.15530234155453,-0.407041111792943,
1.25681160160691));
#34242=CARTESIAN_POINT('Ctrl Pts',(1.10126842659597,-0.387888272594439,
1.30441816675528));
#34243=CARTESIAN_POINT('Ctrl Pts',(1.07446535104584,-0.373243761060364,
1.32643091652006));
#34244=CARTESIAN_POINT('Ctrl Pts',(1.02199477007745,-0.335108247315848,
1.36743459453896));
#34245=CARTESIAN_POINT('Ctrl Pts',(0.990027513266105,-0.303141259068211,
1.39055359345152));
#34246=CARTESIAN_POINT('Ctrl Pts',(0.940896403863071,-0.236152929235937,
1.42432715921571));
#34247=CARTESIAN_POINT('Ctrl Pts',(0.917859913453974,-0.192480977588835,
1.43904931717599));
#34248=CARTESIAN_POINT('Ctrl Pts',(0.895520212222106,-0.123823518623745,
1.45296717977858));
#34249=CARTESIAN_POINT('Ctrl Pts',(0.890059788636851,-0.101649918886749,
1.45630208793976));
#34250=CARTESIAN_POINT('Ctrl Pts',(0.886256117232622,-0.0793800000000001,
1.45861320581289));
#34251=CARTESIAN_POINT('Origin',(1.18440385848747,-0.07938,1.18440385848747));
#34252=CARTESIAN_POINT('Origin',(0.,-0.27783,0.));
#34253=CARTESIAN_POINT('',(0.404717578595295,-0.07938,1.65807299932179));
#34254=CARTESIAN_POINT('Origin',(0.,-0.07938,0.));
#34255=CARTESIAN_POINT('',(-0.404717578595296,-0.07938,1.65807299932179));
#34256=CARTESIAN_POINT('Ctrl Pts',(0.404717578595296,-0.0793800000000001,
1.65807299932179));
#34257=CARTESIAN_POINT('Ctrl Pts',(0.400393769631747,-0.101649918886749,
1.65912839404491));
#34258=CARTESIAN_POINT('Ctrl Pts',(0.394174530911058,-0.123823518623745,
1.66063136041479));
#34259=CARTESIAN_POINT('Ctrl Pts',(0.368536561654407,-0.192480977588835,
1.66658649961961));
#34260=CARTESIAN_POINT('Ctrl Pts',(0.341837165343982,-0.236152929235937,
1.67246562047521));
#34261=CARTESIAN_POINT('Ctrl Pts',(0.283214707341173,-0.303141259068211,
1.68332504372461));
#34262=CARTESIAN_POINT('Ctrl Pts',(0.244262842368623,-0.335108247315849,
1.68958170688653));
#34263=CARTESIAN_POINT('Ctrl Pts',(0.178166559972324,-0.373243761060364,
1.69769003172132));
#34264=CARTESIAN_POINT('Ctrl Pts',(0.143648558862931,-0.387888272594439,
1.70107730356824));
#34265=CARTESIAN_POINT('Ctrl Pts',(0.0717778861362652,-0.407041111792943,
1.70562212620408));
#34266=CARTESIAN_POINT('Ctrl Pts',(0.0344244045173309,-0.411552957311693,
1.706752));
#34267=CARTESIAN_POINT('Ctrl Pts',(-0.0344244045173315,-0.411552957311693,
1.706752));
#34268=CARTESIAN_POINT('Ctrl Pts',(-0.0717778861362658,-0.407041111792943,
1.70562212620408));
#34269=CARTESIAN_POINT('Ctrl Pts',(-0.143648558862932,-0.387888272594439,
1.70107730356824));
#34270=CARTESIAN_POINT('Ctrl Pts',(-0.178166559972325,-0.373243761060364,
1.69769003172132));
#34271=CARTESIAN_POINT('Ctrl Pts',(-0.244262842368624,-0.335108247315849,
1.68958170688653));
#34272=CARTESIAN_POINT('Ctrl Pts',(-0.283214707341173,-0.303141259068212,
1.68332504372461));
#34273=CARTESIAN_POINT('Ctrl Pts',(-0.341837165343982,-0.236152929235937,
1.67246562047521));
#34274=CARTESIAN_POINT('Ctrl Pts',(-0.368536561654408,-0.192480977588835,
1.66658649961961));
#34275=CARTESIAN_POINT('Ctrl Pts',(-0.394174530911059,-0.123823518623745,
1.66063136041479));
#34276=CARTESIAN_POINT('Ctrl Pts',(-0.400393769631748,-0.101649918886749,
1.65912839404491));
#34277=CARTESIAN_POINT('Ctrl Pts',(-0.404717578595297,-0.0793800000000001,
1.65807299932179));
#34278=CARTESIAN_POINT('',(-0.886256117232624,-0.07938,1.45861320581289));
#34279=CARTESIAN_POINT('Origin',(0.,-0.07938,0.));
#34280=CARTESIAN_POINT('',(-1.45861320581289,-0.07938,0.886256117232623));
#34281=CARTESIAN_POINT('Ctrl Pts',(-0.886256117232623,-0.0793800000000001,
1.45861320581289));
#34282=CARTESIAN_POINT('Ctrl Pts',(-0.890059788636852,-0.101649918886749,
1.45630208793976));
#34283=CARTESIAN_POINT('Ctrl Pts',(-0.895520212222106,-0.123823518623745,
1.45296717977858));
#34284=CARTESIAN_POINT('Ctrl Pts',(-0.917859913453974,-0.192480977588835,
1.43904931717599));
#34285=CARTESIAN_POINT('Ctrl Pts',(-0.940896403863071,-0.236152929235937,
1.4243271592157));
#34286=CARTESIAN_POINT('Ctrl Pts',(-0.990027513266105,-0.303141259068211,
1.39055359345152));
#34287=CARTESIAN_POINT('Ctrl Pts',(-1.02199477007745,-0.335108247315848,
1.36743459453896));
#34288=CARTESIAN_POINT('Ctrl Pts',(-1.07446535104584,-0.373243761060364,
1.32643091652006));
#34289=CARTESIAN_POINT('Ctrl Pts',(-1.10126842659597,-0.387888272594439,
1.30441816675528));
#34290=CARTESIAN_POINT('Ctrl Pts',(-1.15530234155453,-0.407041111792943,
1.25681160160691));
#34291=CARTESIAN_POINT('Ctrl Pts',(-1.18251418313119,-0.411552957311693,
1.23119764287622));
#34292=CARTESIAN_POINT('Ctrl Pts',(-1.23119764287622,-0.411552957311693,
1.18251418313119));
#34293=CARTESIAN_POINT('Ctrl Pts',(-1.25681160160691,-0.407041111792943,
1.15530234155453));
#34294=CARTESIAN_POINT('Ctrl Pts',(-1.30441816675528,-0.387888272594439,
1.10126842659597));
#34295=CARTESIAN_POINT('Ctrl Pts',(-1.32643091652006,-0.373243761060365,
1.07446535104584));
#34296=CARTESIAN_POINT('Ctrl Pts',(-1.36743459453896,-0.335108247315849,
1.02199477007745));
#34297=CARTESIAN_POINT('Ctrl Pts',(-1.39055359345152,-0.303141259068212,
0.990027513266106));
#34298=CARTESIAN_POINT('Ctrl Pts',(-1.4243271592157,-0.236152929235938,
0.940896403863071));
#34299=CARTESIAN_POINT('Ctrl Pts',(-1.43904931717599,-0.192480977588836,
0.917859913453974));
#34300=CARTESIAN_POINT('Ctrl Pts',(-1.45296717977858,-0.123823518623746,
0.895520212222106));
#34301=CARTESIAN_POINT('Ctrl Pts',(-1.45630208793976,-0.101649918886749,
0.890059788636852));
#34302=CARTESIAN_POINT('Ctrl Pts',(-1.45861320581289,-0.0793800000000001,
0.886256117232623));
#34303=CARTESIAN_POINT('',(-1.65807299932179,-0.07938,0.404717578595295));
#34304=CARTESIAN_POINT('Origin',(0.,-0.07938,0.));
#34305=CARTESIAN_POINT('',(-1.706752,-0.411552957311693,2.08591827245526E-16));
#34306=CARTESIAN_POINT('Ctrl Pts',(-1.65807299932179,-0.0793800000000001,
0.404717578595296));
#34307=CARTESIAN_POINT('Ctrl Pts',(-1.65912839404491,-0.101649918886749,
0.400393769631747));
#34308=CARTESIAN_POINT('Ctrl Pts',(-1.66063136041479,-0.123823518623745,
0.394174530911058));
#34309=CARTESIAN_POINT('Ctrl Pts',(-1.66658649961961,-0.192480977588835,
0.368536561654407));
#34310=CARTESIAN_POINT('Ctrl Pts',(-1.67246562047521,-0.236152929235937,
0.341837165343982));
#34311=CARTESIAN_POINT('Ctrl Pts',(-1.68332504372461,-0.303141259068211,
0.283214707341173));
#34312=CARTESIAN_POINT('Ctrl Pts',(-1.68958170688653,-0.335108247315848,
0.244262842368623));
#34313=CARTESIAN_POINT('Ctrl Pts',(-1.69769003172132,-0.373243761060364,
0.178166559972324));
#34314=CARTESIAN_POINT('Ctrl Pts',(-1.70107730356824,-0.387888272594439,
0.143648558862931));
#34315=CARTESIAN_POINT('Ctrl Pts',(-1.70562212620408,-0.407041111792943,
0.0717778861362656));
#34316=CARTESIAN_POINT('Ctrl Pts',(-1.706752,-0.411552957311693,0.0344244045173313));
#34317=CARTESIAN_POINT('Ctrl Pts',(-1.706752,-0.411552957311693,2.08166817117217E-16));
#34318=CARTESIAN_POINT('',(-1.706752,-0.47628,2.09016837373834E-16));
#34319=CARTESIAN_POINT('',(-1.706752,-0.27783,2.09016837373834E-16));
#34320=CARTESIAN_POINT('Origin',(0.,-0.47628,0.));
#34321=CARTESIAN_POINT('',(-1.65807299932179,-0.07938,-0.404717578595296));
#34322=CARTESIAN_POINT('Ctrl Pts',(-1.706752,-0.411552957311693,2.0122792321331E-16));
#34323=CARTESIAN_POINT('Ctrl Pts',(-1.706752,-0.411552957311693,-0.0344244045173309));
#34324=CARTESIAN_POINT('Ctrl Pts',(-1.70562212620408,-0.407041111792943,
-0.0717778861362652));
#34325=CARTESIAN_POINT('Ctrl Pts',(-1.70107730356824,-0.387888272594439,
-0.143648558862931));
#34326=CARTESIAN_POINT('Ctrl Pts',(-1.69769003172132,-0.373243761060365,
-0.178166559972324));
#34327=CARTESIAN_POINT('Ctrl Pts',(-1.68958170688653,-0.335108247315849,
-0.244262842368623));
#34328=CARTESIAN_POINT('Ctrl Pts',(-1.68332504372461,-0.303141259068212,
-0.283214707341173));
#34329=CARTESIAN_POINT('Ctrl Pts',(-1.67246562047521,-0.236152929235938,
-0.341837165343982));
#34330=CARTESIAN_POINT('Ctrl Pts',(-1.66658649961961,-0.192480977588836,
-0.368536561654407));
#34331=CARTESIAN_POINT('Ctrl Pts',(-1.66063136041479,-0.123823518623745,
-0.394174530911059));
#34332=CARTESIAN_POINT('Ctrl Pts',(-1.65912839404491,-0.101649918886749,
-0.400393769631748));
#34333=CARTESIAN_POINT('Ctrl Pts',(-1.65807299932179,-0.0793800000000001,
-0.404717578595296));
#34334=CARTESIAN_POINT('',(-1.45861320581289,-0.07938,-0.886256117232623));
#34335=CARTESIAN_POINT('Origin',(0.,-0.07938,0.));
#34336=CARTESIAN_POINT('',(-0.886256117232623,-0.07938,-1.45861320581289));
#34337=CARTESIAN_POINT('Ctrl Pts',(-1.45861320581289,-0.0793800000000001,
-0.886256117232623));
#34338=CARTESIAN_POINT('Ctrl Pts',(-1.45630208793976,-0.101649918886749,
-0.890059788636852));
#34339=CARTESIAN_POINT('Ctrl Pts',(-1.45296717977858,-0.123823518623745,
-0.895520212222106));
#34340=CARTESIAN_POINT('Ctrl Pts',(-1.43904931717599,-0.192480977588835,
-0.917859913453974));
#34341=CARTESIAN_POINT('Ctrl Pts',(-1.4243271592157,-0.236152929235937,
-0.940896403863072));
#34342=CARTESIAN_POINT('Ctrl Pts',(-1.39055359345152,-0.303141259068212,
-0.990027513266106));
#34343=CARTESIAN_POINT('Ctrl Pts',(-1.36743459453896,-0.335108247315849,
-1.02199477007745));
#34344=CARTESIAN_POINT('Ctrl Pts',(-1.32643091652006,-0.373243761060364,
-1.07446535104584));
#34345=CARTESIAN_POINT('Ctrl Pts',(-1.30441816675528,-0.387888272594439,
-1.10126842659597));
#34346=CARTESIAN_POINT('Ctrl Pts',(-1.25681160160691,-0.407041111792943,
-1.15530234155453));
#34347=CARTESIAN_POINT('Ctrl Pts',(-1.23119764287622,-0.411552957311693,
-1.18251418313119));
#34348=CARTESIAN_POINT('Ctrl Pts',(-1.18251418313119,-0.411552957311693,
-1.23119764287622));
#34349=CARTESIAN_POINT('Ctrl Pts',(-1.15530234155453,-0.407041111792943,
-1.25681160160691));
#34350=CARTESIAN_POINT('Ctrl Pts',(-1.10126842659597,-0.387888272594439,
-1.30441816675528));
#34351=CARTESIAN_POINT('Ctrl Pts',(-1.07446535104584,-0.373243761060364,
-1.32643091652006));
#34352=CARTESIAN_POINT('Ctrl Pts',(-1.02199477007745,-0.335108247315848,
-1.36743459453896));
#34353=CARTESIAN_POINT('Ctrl Pts',(-0.990027513266105,-0.303141259068211,
-1.39055359345152));
#34354=CARTESIAN_POINT('Ctrl Pts',(-0.940896403863071,-0.236152929235936,
-1.42432715921571));
#34355=CARTESIAN_POINT('Ctrl Pts',(-0.917859913453974,-0.192480977588835,
-1.43904931717599));
#34356=CARTESIAN_POINT('Ctrl Pts',(-0.895520212222106,-0.123823518623745,
-1.45296717977858));
#34357=CARTESIAN_POINT('Ctrl Pts',(-0.890059788636851,-0.101649918886749,
-1.45630208793976));
#34358=CARTESIAN_POINT('Ctrl Pts',(-0.886256117232623,-0.0793800000000001,
-1.45861320581289));
#34359=CARTESIAN_POINT('',(-0.404717578595295,-0.07938,-1.65807299932179));
#34360=CARTESIAN_POINT('Origin',(0.,-0.07938,0.));
#34361=CARTESIAN_POINT('',(0.404717578595296,-0.07938,-1.65807299932179));
#34362=CARTESIAN_POINT('Ctrl Pts',(-0.404717578595296,-0.0793800000000001,
-1.65807299932179));
#34363=CARTESIAN_POINT('Ctrl Pts',(-0.400393769631747,-0.101649918886749,
-1.65912839404491));
#34364=CARTESIAN_POINT('Ctrl Pts',(-0.394174530911058,-0.123823518623746,
-1.66063136041479));
#34365=CARTESIAN_POINT('Ctrl Pts',(-0.368536561654407,-0.192480977588836,
-1.66658649961961));
#34366=CARTESIAN_POINT('Ctrl Pts',(-0.341837165343982,-0.236152929235938,
-1.67246562047521));
#34367=CARTESIAN_POINT('Ctrl Pts',(-0.283214707341173,-0.303141259068212,
-1.68332504372461));
#34368=CARTESIAN_POINT('Ctrl Pts',(-0.244262842368623,-0.335108247315849,
-1.68958170688653));
#34369=CARTESIAN_POINT('Ctrl Pts',(-0.178166559972324,-0.373243761060364,
-1.69769003172132));
#34370=CARTESIAN_POINT('Ctrl Pts',(-0.143648558862931,-0.387888272594439,
-1.70107730356824));
#34371=CARTESIAN_POINT('Ctrl Pts',(-0.0717778861362653,-0.407041111792943,
-1.70562212620408));
#34372=CARTESIAN_POINT('Ctrl Pts',(-0.034424404517331,-0.411552957311693,
-1.706752));
#34373=CARTESIAN_POINT('Ctrl Pts',(0.0344244045173312,-0.411552957311693,
-1.706752));
#34374=CARTESIAN_POINT('Ctrl Pts',(0.0717778861362655,-0.407041111792943,
-1.70562212620408));
#34375=CARTESIAN_POINT('Ctrl Pts',(0.143648558862931,-0.387888272594439,
-1.70107730356824));
#34376=CARTESIAN_POINT('Ctrl Pts',(0.178166559972324,-0.373243761060364,
-1.69769003172132));
#34377=CARTESIAN_POINT('Ctrl Pts',(0.244262842368623,-0.335108247315849,
-1.68958170688653));
#34378=CARTESIAN_POINT('Ctrl Pts',(0.283214707341173,-0.303141259068212,
-1.68332504372461));
#34379=CARTESIAN_POINT('Ctrl Pts',(0.341837165343982,-0.236152929235937,
-1.67246562047521));
#34380=CARTESIAN_POINT('Ctrl Pts',(0.368536561654407,-0.192480977588835,
-1.66658649961961));
#34381=CARTESIAN_POINT('Ctrl Pts',(0.394174530911059,-0.123823518623745,
-1.66063136041479));
#34382=CARTESIAN_POINT('Ctrl Pts',(0.400393769631748,-0.101649918886749,
-1.65912839404491));
#34383=CARTESIAN_POINT('Ctrl Pts',(0.404717578595296,-0.0793800000000001,
-1.65807299932179));
#34384=CARTESIAN_POINT('',(0.886256117232623,-0.07938,-1.45861320581289));
#34385=CARTESIAN_POINT('Origin',(0.,-0.07938,0.));
#34386=CARTESIAN_POINT('',(1.45861320581289,-0.07938,-0.886256117232623));
#34387=CARTESIAN_POINT('Ctrl Pts',(0.886256117232623,-0.0793800000000001,
-1.45861320581289));
#34388=CARTESIAN_POINT('Ctrl Pts',(0.890059788636852,-0.101649918886749,
-1.45630208793976));
#34389=CARTESIAN_POINT('Ctrl Pts',(0.895520212222106,-0.123823518623745,
-1.45296717977858));
#34390=CARTESIAN_POINT('Ctrl Pts',(0.917859913453974,-0.192480977588835,
-1.43904931717599));
#34391=CARTESIAN_POINT('Ctrl Pts',(0.940896403863072,-0.236152929235937,
-1.4243271592157));
#34392=CARTESIAN_POINT('Ctrl Pts',(0.990027513266106,-0.303141259068211,
-1.39055359345152));
#34393=CARTESIAN_POINT('Ctrl Pts',(1.02199477007745,-0.335108247315849,
-1.36743459453896));
#34394=CARTESIAN_POINT('Ctrl Pts',(1.07446535104584,-0.373243761060364,
-1.32643091652006));
#34395=CARTESIAN_POINT('Ctrl Pts',(1.10126842659597,-0.387888272594439,
-1.30441816675528));
#34396=CARTESIAN_POINT('Ctrl Pts',(1.15530234155453,-0.407041111792943,
-1.25681160160691));
#34397=CARTESIAN_POINT('Ctrl Pts',(1.18251418313119,-0.411552957311693,
-1.23119764287622));
#34398=CARTESIAN_POINT('Ctrl Pts',(1.23119764287622,-0.411552957311693,
-1.18251418313119));
#34399=CARTESIAN_POINT('Ctrl Pts',(1.25681160160691,-0.407041111792943,
-1.15530234155453));
#34400=CARTESIAN_POINT('Ctrl Pts',(1.30441816675528,-0.387888272594439,
-1.10126842659597));
#34401=CARTESIAN_POINT('Ctrl Pts',(1.32643091652006,-0.373243761060364,
-1.07446535104584));
#34402=CARTESIAN_POINT('Ctrl Pts',(1.36743459453896,-0.335108247315849,
-1.02199477007745));
#34403=CARTESIAN_POINT('Ctrl Pts',(1.39055359345152,-0.303141259068212,
-0.990027513266105));
#34404=CARTESIAN_POINT('Ctrl Pts',(1.4243271592157,-0.236152929235937,-0.940896403863071));
#34405=CARTESIAN_POINT('Ctrl Pts',(1.43904931717599,-0.192480977588835,
-0.917859913453974));
#34406=CARTESIAN_POINT('Ctrl Pts',(1.45296717977858,-0.123823518623745,
-0.895520212222106));
#34407=CARTESIAN_POINT('Ctrl Pts',(1.45630208793976,-0.101649918886749,
-0.890059788636852));
#34408=CARTESIAN_POINT('Ctrl Pts',(1.45861320581289,-0.0793800000000001,
-0.886256117232623));
#34409=CARTESIAN_POINT('',(1.65807299932179,-0.07938,-0.404717578595296));
#34410=CARTESIAN_POINT('Origin',(0.,-0.07938,0.));
#34411=CARTESIAN_POINT('',(1.65807299932179,-0.07938,0.404717578595296));
#34412=CARTESIAN_POINT('Ctrl Pts',(1.65807299932179,-0.0793800000000001,
-0.404717578595296));
#34413=CARTESIAN_POINT('Ctrl Pts',(1.65912839404491,-0.101649918886749,
-0.400393769631747));
#34414=CARTESIAN_POINT('Ctrl Pts',(1.66063136041479,-0.123823518623745,
-0.394174530911058));
#34415=CARTESIAN_POINT('Ctrl Pts',(1.66658649961961,-0.192480977588835,
-0.368536561654407));
#34416=CARTESIAN_POINT('Ctrl Pts',(1.67246562047521,-0.236152929235937,
-0.341837165343982));
#34417=CARTESIAN_POINT('Ctrl Pts',(1.68332504372461,-0.303141259068212,
-0.283214707341173));
#34418=CARTESIAN_POINT('Ctrl Pts',(1.68958170688653,-0.335108247315849,
-0.244262842368623));
#34419=CARTESIAN_POINT('Ctrl Pts',(1.69769003172132,-0.373243761060364,
-0.178166559972324));
#34420=CARTESIAN_POINT('Ctrl Pts',(1.70107730356824,-0.387888272594439,
-0.143648558862931));
#34421=CARTESIAN_POINT('Ctrl Pts',(1.70562212620408,-0.407041111792943,
-0.0717778861362655));
#34422=CARTESIAN_POINT('Ctrl Pts',(1.706752,-0.411552957311693,-0.0344244045173312));
#34423=CARTESIAN_POINT('Ctrl Pts',(1.706752,-0.411552957311693,0.0344244045173312));
#34424=CARTESIAN_POINT('Ctrl Pts',(1.70562212620408,-0.407041111792943,
0.0717778861362655));
#34425=CARTESIAN_POINT('Ctrl Pts',(1.70107730356824,-0.387888272594439,
0.143648558862931));
#34426=CARTESIAN_POINT('Ctrl Pts',(1.69769003172132,-0.373243761060364,
0.178166559972324));
#34427=CARTESIAN_POINT('Ctrl Pts',(1.68958170688653,-0.335108247315849,
0.244262842368623));
#34428=CARTESIAN_POINT('Ctrl Pts',(1.68332504372461,-0.303141259068212,
0.283214707341173));
#34429=CARTESIAN_POINT('Ctrl Pts',(1.67246562047521,-0.236152929235937,
0.341837165343982));
#34430=CARTESIAN_POINT('Ctrl Pts',(1.66658649961961,-0.192480977588835,
0.368536561654407));
#34431=CARTESIAN_POINT('Ctrl Pts',(1.66063136041479,-0.123823518623745,
0.394174530911058));
#34432=CARTESIAN_POINT('Ctrl Pts',(1.65912839404491,-0.101649918886749,
0.400393769631747));
#34433=CARTESIAN_POINT('Ctrl Pts',(1.65807299932179,-0.0793800000000001,
0.404717578595296));
#34434=CARTESIAN_POINT('Origin',(0.,-0.07938,0.));
#34435=CARTESIAN_POINT('Origin',(0.,-0.07938,0.));
#34436=CARTESIAN_POINT('',(0.397005914195118,-0.07938,1.59456899932179));
#34437=CARTESIAN_POINT('Origin',(0.,-0.07938,0.));
#34438=CARTESIAN_POINT('Origin',(-3.33066907387547E-16,-0.07938,1.675));
#34439=CARTESIAN_POINT('Origin',(-3.33066907387547E-16,0.,1.675));
#34440=CARTESIAN_POINT('',(-0.397005914195118,-0.07938,1.59456899932179));
#34441=CARTESIAN_POINT('Ctrl Pts',(-0.397005914195119,-0.0793800000000001,
1.59456899932179));
#34442=CARTESIAN_POINT('Ctrl Pts',(-0.3886265584581,-0.123401821157026,
1.59665523941937));
#34443=CARTESIAN_POINT('Ctrl Pts',(-0.373030350867485,-0.166543350814306,
1.60050712143809));
#34444=CARTESIAN_POINT('Ctrl Pts',(-0.333298652394954,-0.237231147975234,
1.60919314384089));
#34445=CARTESIAN_POINT('Ctrl Pts',(-0.311480544243687,-0.266264900654909,
1.61365775139403));
#34446=CARTESIAN_POINT('Ctrl Pts',(-0.261368388670537,-0.317195968905306,
1.62252828437015));
#34447=CARTESIAN_POINT('Ctrl Pts',(-0.233069203882014,-0.33909093068465,
1.62691869420078));
#34448=CARTESIAN_POINT('Ctrl Pts',(-0.174042761838764,-0.373586846396559,
1.63426473152765));
#34449=CARTESIAN_POINT('Ctrl Pts',(-0.14036578147155,-0.388086240756494,
1.63761964365402));
#34450=CARTESIAN_POINT('Ctrl Pts',(-0.0701778381840615,-0.407068917407805,
1.64212536811722));
#34451=CARTESIAN_POINT('Ctrl Pts',(-0.0336652739555918,-0.411552957311693,
1.643248));
#34452=CARTESIAN_POINT('Ctrl Pts',(0.0336652739555913,-0.411552957311693,
1.643248));
#34453=CARTESIAN_POINT('Ctrl Pts',(0.070177838184061,-0.407068917407805,
1.64212536811722));
#34454=CARTESIAN_POINT('Ctrl Pts',(0.140365781471549,-0.388086240756494,
1.63761964365402));
#34455=CARTESIAN_POINT('Ctrl Pts',(0.174042761838763,-0.373586846396559,
1.63426473152765));
#34456=CARTESIAN_POINT('Ctrl Pts',(0.233069203882014,-0.33909093068465,
1.62691869420078));
#34457=CARTESIAN_POINT('Ctrl Pts',(0.261368388670536,-0.317195968905306,
1.62252828437015));
#34458=CARTESIAN_POINT('Ctrl Pts',(0.311480544243686,-0.266264900654908,
1.61365775139403));
#34459=CARTESIAN_POINT('Ctrl Pts',(0.333298652394954,-0.237231147975234,
1.60919314384089));
#34460=CARTESIAN_POINT('Ctrl Pts',(0.373030350867484,-0.166543350814306,
1.60050712143809));
#34461=CARTESIAN_POINT('Ctrl Pts',(0.388626558458099,-0.123401821157026,
1.59665523941937));
#34462=CARTESIAN_POINT('Ctrl Pts',(0.397005914195118,-0.07938,1.59456899932179));
#34463=CARTESIAN_POINT('Origin',(-3.33066907387547E-16,-0.07938,1.675));
#34464=CARTESIAN_POINT('Origin',(0.,-0.07938,0.));
#34465=CARTESIAN_POINT('',(-0.846804978391754,-0.07938,1.40825612658882));
#34466=CARTESIAN_POINT('Origin',(0.,-0.07938,0.));
#34467=CARTESIAN_POINT('Origin',(-1.18440385848747,-0.07938,1.18440385848747));
#34468=CARTESIAN_POINT('Origin',(-1.18440385848747,0.,1.18440385848747));
#34469=CARTESIAN_POINT('',(-1.40825612658882,-0.07938,0.846804978391753));
#34470=CARTESIAN_POINT('Ctrl Pts',(-1.40825612658882,-0.0793800000000001,
0.846804978391753));
#34471=CARTESIAN_POINT('Ctrl Pts',(-1.40380622184538,-0.123401821157026,
0.854205272175555));
#34472=CARTESIAN_POINT('Ctrl Pts',(-1.39550172959303,-0.166543350814306,
0.867957148219442));
#34473=CARTESIAN_POINT('Ctrl Pts',(-1.3735491215176,-0.237231147975235,
0.902193646979983));
#34474=CARTESIAN_POINT('Ctrl Pts',(-1.36127834356734,-0.266264900654909,
0.920778333482565));
#34475=CARTESIAN_POINT('Ctrl Pts',(-1.33211611256184,-0.317195968905306,
0.962485392528369));
#34476=CARTESIAN_POINT('Ctrl Pts',(-1.31521005565926,-0.339090930684651,
0.985600426557816));
#34477=CARTESIAN_POINT('Ctrl Pts',(-1.27866649102984,-0.373586846396559,
1.03253285680459));
#34478=CARTESIAN_POINT('Ctrl Pts',(-1.25722555095714,-0.388086240756494,
1.05871835910697));
#34479=CARTESIAN_POINT('Ctrl Pts',(-1.2107812086231,-0.407068917407805,
1.11153475808518));
#34480=CARTESIAN_POINT('Ctrl Pts',(-1.18575674747573,-0.411552957311693,
1.13814686046673));
#34481=CARTESIAN_POINT('Ctrl Pts',(-1.13814686046673,-0.411552957311693,
1.18575674747573));
#34482=CARTESIAN_POINT('Ctrl Pts',(-1.11153475808518,-0.407068917407805,
1.2107812086231));
#34483=CARTESIAN_POINT('Ctrl Pts',(-1.05871835910697,-0.388086240756494,
1.25722555095714));
#34484=CARTESIAN_POINT('Ctrl Pts',(-1.03253285680459,-0.373586846396559,
1.27866649102984));
#34485=CARTESIAN_POINT('Ctrl Pts',(-0.985600426557816,-0.33909093068465,
1.31521005565926));
#34486=CARTESIAN_POINT('Ctrl Pts',(-0.962485392528369,-0.317195968905306,
1.33211611256184));
#34487=CARTESIAN_POINT('Ctrl Pts',(-0.920778333482565,-0.266264900654908,
1.36127834356734));
#34488=CARTESIAN_POINT('Ctrl Pts',(-0.902193646979983,-0.237231147975234,
1.3735491215176));
#34489=CARTESIAN_POINT('Ctrl Pts',(-0.867957148219442,-0.166543350814306,
1.39550172959303));
#34490=CARTESIAN_POINT('Ctrl Pts',(-0.854205272175555,-0.123401821157026,
1.40380622184538));
#34491=CARTESIAN_POINT('Ctrl Pts',(-0.846804978391753,-0.0793800000000001,
1.40825612658882));
#34492=CARTESIAN_POINT('Origin',(-1.18440385848747,-0.07938,1.18440385848747));
#34493=CARTESIAN_POINT('Origin',(0.,-0.07938,0.));
#34494=CARTESIAN_POINT('',(-1.59456899932179,-0.07938,0.397005914195118));
#34495=CARTESIAN_POINT('Origin',(0.,-0.07938,0.));
#34496=CARTESIAN_POINT('Origin',(-1.675,-0.07938,-2.22044604925031E-16));
#34497=CARTESIAN_POINT('Origin',(-1.675,0.,-2.22044604925031E-16));
#34498=CARTESIAN_POINT('',(-1.59456899932179,-0.07938,-0.397005914195118));
#34499=CARTESIAN_POINT('',(-1.643248,-0.411552957311693,3.47540551556327E-18));
#34500=CARTESIAN_POINT('Ctrl Pts',(-1.59456899932179,-0.0793800000000001,
-0.397005914195119));
#34501=CARTESIAN_POINT('Ctrl Pts',(-1.59665523941937,-0.123401821157026,
-0.388626558458099));
#34502=CARTESIAN_POINT('Ctrl Pts',(-1.60050712143809,-0.166543350814306,
-0.373030350867485));
#34503=CARTESIAN_POINT('Ctrl Pts',(-1.60919314384089,-0.237231147975234,
-0.333298652394954));
#34504=CARTESIAN_POINT('Ctrl Pts',(-1.61365775139403,-0.266264900654909,
-0.311480544243686));
#34505=CARTESIAN_POINT('Ctrl Pts',(-1.62252828437015,-0.317195968905306,
-0.261368388670537));
#34506=CARTESIAN_POINT('Ctrl Pts',(-1.62691869420078,-0.33909093068465,
-0.233069203882014));
#34507=CARTESIAN_POINT('Ctrl Pts',(-1.63426473152765,-0.373586846396559,
-0.174042761838764));
#34508=CARTESIAN_POINT('Ctrl Pts',(-1.63761964365402,-0.388086240756494,
-0.140365781471549));
#34509=CARTESIAN_POINT('Ctrl Pts',(-1.64212536811722,-0.407068917407805,
-0.0701778381840614));
#34510=CARTESIAN_POINT('Ctrl Pts',(-1.643248,-0.411552957311693,-0.0336652739555917));
#34511=CARTESIAN_POINT('Ctrl Pts',(-1.643248,-0.411552957311693,-2.0122792321331E-16));
#34512=CARTESIAN_POINT('Origin',(-1.675,-0.07938,-2.22044604925031E-16));
#34513=CARTESIAN_POINT('Ctrl Pts',(-1.643248,-0.411552957311693,-1.94289029309402E-16));
#34514=CARTESIAN_POINT('Ctrl Pts',(-1.643248,-0.411552957311693,0.0336652739555913));
#34515=CARTESIAN_POINT('Ctrl Pts',(-1.64212536811722,-0.407068917407805,
0.0701778381840609));
#34516=CARTESIAN_POINT('Ctrl Pts',(-1.63761964365402,-0.388086240756494,
0.140365781471549));
#34517=CARTESIAN_POINT('Ctrl Pts',(-1.63426473152765,-0.373586846396559,
0.174042761838763));
#34518=CARTESIAN_POINT('Ctrl Pts',(-1.62691869420078,-0.33909093068465,
0.233069203882014));
#34519=CARTESIAN_POINT('Ctrl Pts',(-1.62252828437015,-0.317195968905306,
0.261368388670536));
#34520=CARTESIAN_POINT('Ctrl Pts',(-1.61365775139403,-0.266264900654909,
0.311480544243686));
#34521=CARTESIAN_POINT('Ctrl Pts',(-1.60919314384089,-0.237231147975235,
0.333298652394954));
#34522=CARTESIAN_POINT('Ctrl Pts',(-1.60050712143809,-0.166543350814306,
0.373030350867484));
#34523=CARTESIAN_POINT('Ctrl Pts',(-1.59665523941937,-0.123401821157026,
0.388626558458099));
#34524=CARTESIAN_POINT('Ctrl Pts',(-1.59456899932179,-0.0793800000000001,
0.397005914195118));
#34525=CARTESIAN_POINT('Origin',(0.,-0.07938,0.));
#34526=CARTESIAN_POINT('',(-1.40825612658882,-0.07938,-0.846804978391753));
#34527=CARTESIAN_POINT('Origin',(0.,-0.07938,0.));
#34528=CARTESIAN_POINT('Origin',(-1.18440385848747,-0.07938,-1.18440385848747));
#34529=CARTESIAN_POINT('Origin',(-1.18440385848747,0.,-1.18440385848747));
#34530=CARTESIAN_POINT('',(-0.846804978391753,-0.07938,-1.40825612658882));
#34531=CARTESIAN_POINT('Ctrl Pts',(-0.846804978391753,-0.0793800000000001,
-1.40825612658882));
#34532=CARTESIAN_POINT('Ctrl Pts',(-0.854205272175555,-0.123401821157026,
-1.40380622184538));
#34533=CARTESIAN_POINT('Ctrl Pts',(-0.867957148219442,-0.166543350814306,
-1.39550172959303));
#34534=CARTESIAN_POINT('Ctrl Pts',(-0.902193646979982,-0.237231147975234,
-1.3735491215176));
#34535=CARTESIAN_POINT('Ctrl Pts',(-0.920778333482564,-0.266264900654908,
-1.36127834356734));
#34536=CARTESIAN_POINT('Ctrl Pts',(-0.962485392528368,-0.317195968905306,
-1.33211611256184));
#34537=CARTESIAN_POINT('Ctrl Pts',(-0.985600426557816,-0.33909093068465,
-1.31521005565926));
#34538=CARTESIAN_POINT('Ctrl Pts',(-1.03253285680459,-0.373586846396559,
-1.27866649102984));
#34539=CARTESIAN_POINT('Ctrl Pts',(-1.05871835910697,-0.388086240756494,
-1.25722555095714));
#34540=CARTESIAN_POINT('Ctrl Pts',(-1.11153475808518,-0.407068917407805,
-1.2107812086231));
#34541=CARTESIAN_POINT('Ctrl Pts',(-1.13814686046673,-0.411552957311693,
-1.18575674747573));
#34542=CARTESIAN_POINT('Ctrl Pts',(-1.18575674747573,-0.411552957311693,
-1.13814686046673));
#34543=CARTESIAN_POINT('Ctrl Pts',(-1.2107812086231,-0.407068917407805,
-1.11153475808518));
#34544=CARTESIAN_POINT('Ctrl Pts',(-1.25722555095714,-0.388086240756494,
-1.05871835910697));
#34545=CARTESIAN_POINT('Ctrl Pts',(-1.27866649102984,-0.373586846396559,
-1.03253285680459));
#34546=CARTESIAN_POINT('Ctrl Pts',(-1.31521005565926,-0.33909093068465,
-0.985600426557816));
#34547=CARTESIAN_POINT('Ctrl Pts',(-1.33211611256184,-0.317195968905306,
-0.962485392528369));
#34548=CARTESIAN_POINT('Ctrl Pts',(-1.36127834356734,-0.266264900654909,
-0.920778333482565));
#34549=CARTESIAN_POINT('Ctrl Pts',(-1.3735491215176,-0.237231147975234,
-0.902193646979983));
#34550=CARTESIAN_POINT('Ctrl Pts',(-1.39550172959303,-0.166543350814306,
-0.867957148219442));
#34551=CARTESIAN_POINT('Ctrl Pts',(-1.40380622184538,-0.123401821157026,
-0.854205272175555));
#34552=CARTESIAN_POINT('Ctrl Pts',(-1.40825612658882,-0.07938,-0.846804978391753));
#34553=CARTESIAN_POINT('Origin',(-1.18440385848747,-0.07938,-1.18440385848747));
#34554=CARTESIAN_POINT('Origin',(0.,-0.07938,0.));
#34555=CARTESIAN_POINT('',(-0.397005914195118,-0.07938,-1.59456899932179));
#34556=CARTESIAN_POINT('Origin',(0.,-0.07938,0.));
#34557=CARTESIAN_POINT('Origin',(1.11022302462516E-16,-0.07938,-1.675));
#34558=CARTESIAN_POINT('Origin',(1.11022302462516E-16,0.,-1.675));
#34559=CARTESIAN_POINT('',(0.397005914195118,-0.07938,-1.59456899932179));
#34560=CARTESIAN_POINT('Ctrl Pts',(0.397005914195119,-0.0793800000000001,
-1.59456899932179));
#34561=CARTESIAN_POINT('Ctrl Pts',(0.388626558458099,-0.123401821157026,
-1.59665523941937));
#34562=CARTESIAN_POINT('Ctrl Pts',(0.373030350867485,-0.166543350814306,
-1.60050712143809));
#34563=CARTESIAN_POINT('Ctrl Pts',(0.333298652394954,-0.237231147975234,
-1.60919314384089));
#34564=CARTESIAN_POINT('Ctrl Pts',(0.311480544243686,-0.266264900654909,
-1.61365775139403));
#34565=CARTESIAN_POINT('Ctrl Pts',(0.261368388670537,-0.317195968905306,
-1.62252828437015));
#34566=CARTESIAN_POINT('Ctrl Pts',(0.233069203882014,-0.33909093068465,
-1.62691869420078));
#34567=CARTESIAN_POINT('Ctrl Pts',(0.174042761838763,-0.373586846396559,
-1.63426473152765));
#34568=CARTESIAN_POINT('Ctrl Pts',(0.140365781471549,-0.388086240756494,
-1.63761964365402));
#34569=CARTESIAN_POINT('Ctrl Pts',(0.0701778381840612,-0.407068917407805,
-1.64212536811722));
#34570=CARTESIAN_POINT('Ctrl Pts',(0.0336652739555916,-0.411552957311693,
-1.643248));
#34571=CARTESIAN_POINT('Ctrl Pts',(-0.0336652739555915,-0.411552957311693,
-1.643248));
#34572=CARTESIAN_POINT('Ctrl Pts',(-0.0701778381840612,-0.407068917407805,
-1.64212536811722));
#34573=CARTESIAN_POINT('Ctrl Pts',(-0.140365781471549,-0.388086240756494,
-1.63761964365402));
#34574=CARTESIAN_POINT('Ctrl Pts',(-0.174042761838764,-0.373586846396559,
-1.63426473152765));
#34575=CARTESIAN_POINT('Ctrl Pts',(-0.233069203882014,-0.33909093068465,
-1.62691869420078));
#34576=CARTESIAN_POINT('Ctrl Pts',(-0.261368388670536,-0.317195968905306,
-1.62252828437015));
#34577=CARTESIAN_POINT('Ctrl Pts',(-0.311480544243686,-0.266264900654908,
-1.61365775139403));
#34578=CARTESIAN_POINT('Ctrl Pts',(-0.333298652394954,-0.237231147975234,
-1.60919314384089));
#34579=CARTESIAN_POINT('Ctrl Pts',(-0.373030350867485,-0.166543350814306,
-1.60050712143809));
#34580=CARTESIAN_POINT('Ctrl Pts',(-0.388626558458099,-0.123401821157026,
-1.59665523941937));
#34581=CARTESIAN_POINT('Ctrl Pts',(-0.397005914195118,-0.07938,-1.59456899932179));
#34582=CARTESIAN_POINT('Origin',(1.11022302462516E-16,-0.07938,-1.675));
#34583=CARTESIAN_POINT('Origin',(0.,-0.07938,0.));
#34584=CARTESIAN_POINT('',(0.846804978391753,-0.07938,-1.40825612658882));
#34585=CARTESIAN_POINT('Origin',(0.,-0.07938,0.));
#34586=CARTESIAN_POINT('Origin',(1.18440385848747,-0.07938,-1.18440385848747));
#34587=CARTESIAN_POINT('Origin',(1.18440385848747,0.,-1.18440385848747));
#34588=CARTESIAN_POINT('',(1.40825612658882,-0.07938,-0.846804978391753));
#34589=CARTESIAN_POINT('Ctrl Pts',(1.40825612658882,-0.0793800000000001,
-0.846804978391753));
#34590=CARTESIAN_POINT('Ctrl Pts',(1.40380622184538,-0.123401821157026,
-0.854205272175555));
#34591=CARTESIAN_POINT('Ctrl Pts',(1.39550172959303,-0.166543350814306,
-0.867957148219442));
#34592=CARTESIAN_POINT('Ctrl Pts',(1.3735491215176,-0.237231147975234,-0.902193646979983));
#34593=CARTESIAN_POINT('Ctrl Pts',(1.36127834356734,-0.266264900654908,
-0.920778333482565));
#34594=CARTESIAN_POINT('Ctrl Pts',(1.33211611256184,-0.317195968905306,
-0.962485392528369));
#34595=CARTESIAN_POINT('Ctrl Pts',(1.31521005565926,-0.33909093068465,-0.985600426557816));
#34596=CARTESIAN_POINT('Ctrl Pts',(1.27866649102984,-0.373586846396559,
-1.03253285680459));
#34597=CARTESIAN_POINT('Ctrl Pts',(1.25722555095714,-0.388086240756494,
-1.05871835910697));
#34598=CARTESIAN_POINT('Ctrl Pts',(1.2107812086231,-0.407068917407805,-1.11153475808518));
#34599=CARTESIAN_POINT('Ctrl Pts',(1.18575674747573,-0.411552957311693,
-1.13814686046673));
#34600=CARTESIAN_POINT('Ctrl Pts',(1.13814686046673,-0.411552957311693,
-1.18575674747573));
#34601=CARTESIAN_POINT('Ctrl Pts',(1.11153475808518,-0.407068917407805,
-1.2107812086231));
#34602=CARTESIAN_POINT('Ctrl Pts',(1.05871835910697,-0.388086240756494,
-1.25722555095714));
#34603=CARTESIAN_POINT('Ctrl Pts',(1.03253285680459,-0.373586846396559,
-1.27866649102984));
#34604=CARTESIAN_POINT('Ctrl Pts',(0.985600426557816,-0.33909093068465,
-1.31521005565926));
#34605=CARTESIAN_POINT('Ctrl Pts',(0.962485392528369,-0.317195968905306,
-1.33211611256184));
#34606=CARTESIAN_POINT('Ctrl Pts',(0.920778333482565,-0.266264900654909,
-1.36127834356734));
#34607=CARTESIAN_POINT('Ctrl Pts',(0.902193646979983,-0.237231147975234,
-1.3735491215176));
#34608=CARTESIAN_POINT('Ctrl Pts',(0.867957148219442,-0.166543350814306,
-1.39550172959303));
#34609=CARTESIAN_POINT('Ctrl Pts',(0.854205272175555,-0.123401821157026,
-1.40380622184538));
#34610=CARTESIAN_POINT('Ctrl Pts',(0.846804978391753,-0.0793800000000001,
-1.40825612658882));
#34611=CARTESIAN_POINT('Origin',(1.18440385848747,-0.07938,-1.18440385848747));
#34612=CARTESIAN_POINT('Origin',(0.,-0.27783,0.));
#34613=CARTESIAN_POINT('',(-1.643248,-0.47628,2.01239840340529E-16));
#34614=CARTESIAN_POINT('Origin',(0.,-0.47628,0.));
#34615=CARTESIAN_POINT('',(-1.643248,-0.27783,2.01239840340529E-16));
#34616=CARTESIAN_POINT('',(1.59456899932179,-0.07938,0.397005914195118));
#34617=CARTESIAN_POINT('Origin',(0.,-0.07938,0.));
#34618=CARTESIAN_POINT('',(1.59456899932179,-0.07938,-0.397005914195118));
#34619=CARTESIAN_POINT('Ctrl Pts',(1.59456899932179,-0.0793800000000001,
0.397005914195118));
#34620=CARTESIAN_POINT('Ctrl Pts',(1.59665523941937,-0.123401821157026,
0.388626558458099));
#34621=CARTESIAN_POINT('Ctrl Pts',(1.60050712143809,-0.166543350814306,
0.373030350867485));
#34622=CARTESIAN_POINT('Ctrl Pts',(1.60919314384089,-0.237231147975234,
0.333298652394954));
#34623=CARTESIAN_POINT('Ctrl Pts',(1.61365775139403,-0.266264900654909,
0.311480544243686));
#34624=CARTESIAN_POINT('Ctrl Pts',(1.62252828437015,-0.317195968905306,
0.261368388670537));
#34625=CARTESIAN_POINT('Ctrl Pts',(1.62691869420078,-0.33909093068465,0.233069203882014));
#34626=CARTESIAN_POINT('Ctrl Pts',(1.63426473152765,-0.373586846396559,
0.174042761838764));
#34627=CARTESIAN_POINT('Ctrl Pts',(1.63761964365402,-0.388086240756494,
0.140365781471549));
#34628=CARTESIAN_POINT('Ctrl Pts',(1.64212536811722,-0.407068917407805,
0.0701778381840612));
#34629=CARTESIAN_POINT('Ctrl Pts',(1.643248,-0.411552957311693,0.0336652739555916));
#34630=CARTESIAN_POINT('Ctrl Pts',(1.643248,-0.411552957311693,-0.0336652739555916));
#34631=CARTESIAN_POINT('Ctrl Pts',(1.64212536811722,-0.407068917407805,
-0.0701778381840612));
#34632=CARTESIAN_POINT('Ctrl Pts',(1.63761964365402,-0.388086240756494,
-0.140365781471549));
#34633=CARTESIAN_POINT('Ctrl Pts',(1.63426473152765,-0.373586846396559,
-0.174042761838764));
#34634=CARTESIAN_POINT('Ctrl Pts',(1.62691869420078,-0.33909093068465,-0.233069203882014));
#34635=CARTESIAN_POINT('Ctrl Pts',(1.62252828437015,-0.317195968905306,
-0.261368388670537));
#34636=CARTESIAN_POINT('Ctrl Pts',(1.61365775139403,-0.266264900654909,
-0.311480544243686));
#34637=CARTESIAN_POINT('Ctrl Pts',(1.60919314384089,-0.237231147975234,
-0.333298652394954));
#34638=CARTESIAN_POINT('Ctrl Pts',(1.60050712143809,-0.166543350814306,
-0.373030350867485));
#34639=CARTESIAN_POINT('Ctrl Pts',(1.59665523941937,-0.123401821157026,
-0.388626558458099));
#34640=CARTESIAN_POINT('Ctrl Pts',(1.59456899932179,-0.07938,-0.397005914195118));
#34641=CARTESIAN_POINT('Origin',(0.,-0.07938,0.));
#34642=CARTESIAN_POINT('Origin',(0.,-0.07938,0.));
#34643=CARTESIAN_POINT('Origin',(1.675,-0.07938,0.));
#34644=CARTESIAN_POINT('Origin',(1.675,0.,0.));
#34645=CARTESIAN_POINT('Origin',(1.675,-0.07938,0.));
#34646=CARTESIAN_POINT('Origin',(0.,-0.47628,0.));
#34647=CARTESIAN_POINT('Origin',(0.,-0.07938,0.));
#62811=UNCERTAINTY_MEASURE_WITH_UNIT(LENGTH_MEASURE(0.001),#62985,
'DISTANCE_ACCURACY_VALUE',
'Maximum model space distance between geometric entities at asserted c
onnectivities');
#62885=UNCERTAINTY_MEASURE_WITH_UNIT(LENGTH_MEASURE(0.001),#62985,
'DISTANCE_ACCURACY_VALUE',
'Maximum model space distance between geometric entities at asserted c
onnectivities');
#62910=(
GEOMETRIC_REPRESENTATION_CONTEXT(3)
GLOBAL_UNCERTAINTY_ASSIGNED_CONTEXT((#62811))
GLOBAL_UNIT_ASSIGNED_CONTEXT((#62985,#62987,#62988))
REPRESENTATION_CONTEXT('','3D')
);
#62984=(
GEOMETRIC_REPRESENTATION_CONTEXT(3)
GLOBAL_UNCERTAINTY_ASSIGNED_CONTEXT((#62885))
GLOBAL_UNIT_ASSIGNED_CONTEXT((#62985,#62987,#62988))
REPRESENTATION_CONTEXT('','3D')
);
#62985=(
LENGTH_UNIT()
NAMED_UNIT(*)
SI_UNIT(.CENTI.,.METRE.)
);
#62987=(
NAMED_UNIT(*)
PLANE_ANGLE_UNIT()
SI_UNIT($,.RADIAN.)
);
#62988=(
NAMED_UNIT(*)
SI_UNIT($,.STERADIAN.)
SOLID_ANGLE_UNIT()
);
#63013=SHAPE_DEFINITION_REPRESENTATION(#63116,#63373);
#63116=PRODUCT_DEFINITION_SHAPE('',$,#63472);
#63373=SHAPE_REPRESENTATION('',(#24471),#62910);
#63447=PRODUCT_DEFINITION_CONTEXT('part definition',#63743,'design');
#63472=PRODUCT_DEFINITION('Cage (1)','Cage (1)',#63570,#63447);
#63570=PRODUCT_DEFINITION_FORMATION('',$,#63769);
#63743=APPLICATION_CONTEXT(
'Core Data for Automotive Mechanical Design Process');
#63744=PRODUCT_CONTEXT('part definition',#63743,'mechanical');
#63769=PRODUCT('Cage (1)','Cage (1)','Cage (1)',(#63744));
#63906=COLOUR_RGB('Grey',0.48,0.52,0.57);
#63907=FILL_AREA_STYLE_COLOUR('',#63906);
#63908=FILL_AREA_STYLE('',(#63907));
#63909=SURFACE_STYLE_FILL_AREA(#63908);
#63910=SURFACE_SIDE_STYLE('',(#63909));
#63911=SURFACE_STYLE_USAGE(.BOTH.,#63910);
#63912=PRESENTATION_STYLE_ASSIGNMENT((#63911));
ENDSEC;
END-ISO-10303-21;
